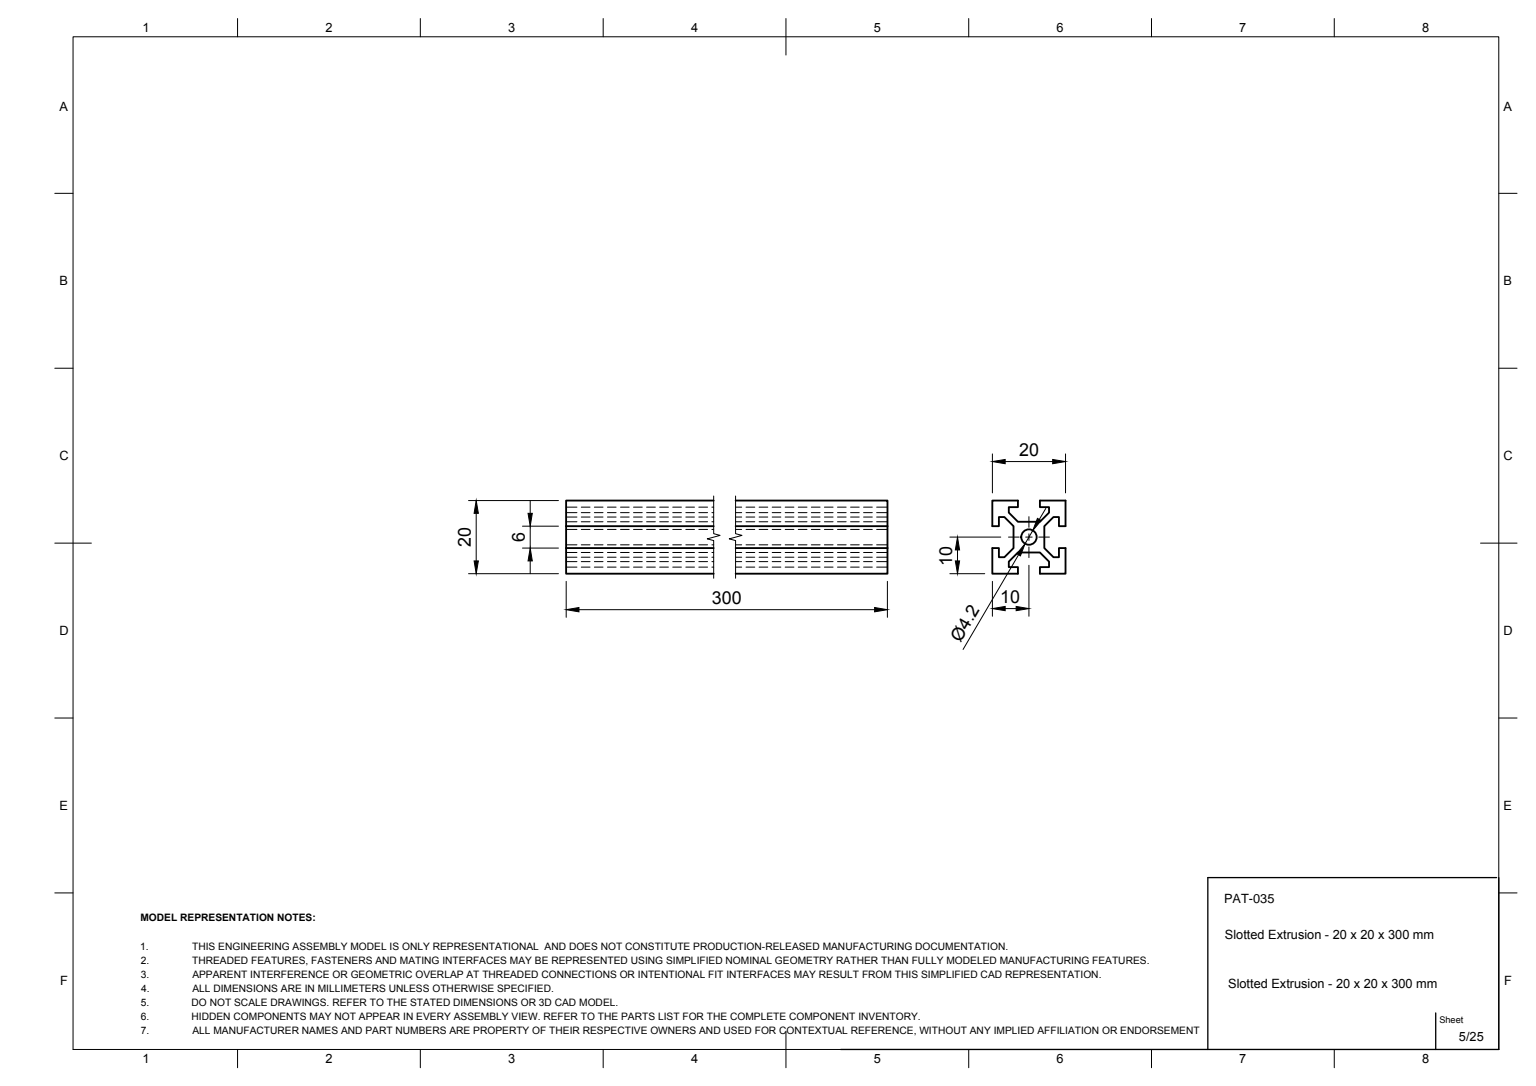
ISO-10303-21;
HEADER;
/* Generated by software containing ST-Developer
 * from STEP Tools, Inc. (www.steptools.com) 
 */

FILE_DESCRIPTION(
/* description */ ('Five-roller gravity conveyor'),
/* implementation_level */ '2;1');

FILE_NAME(
/* name */ 'Slotted Extrusion - 20 x 20 x 300 mm.step',
/* time_stamp */ '2026-10-29T15:36:43-07:00',
/* author */ (''),
/* organization */ (''),
/* preprocessor_version */ 'ST-DEVELOPER v20.2',
/* originating_system */ 'Autodesk Translation Framework v15.17.0.0',
/* authorisation */ '');

FILE_SCHEMA (('AUTOMOTIVE_DESIGN { 1 0 10303 214 3 1 1 }'));
ENDSEC;

DATA;
#10=MECHANICAL_DESIGN_GEOMETRIC_PRESENTATION_REPRESENTATION('',(#312),#7806);
#276=SHAPE_REPRESENTATION_RELATIONSHIP('SRR','None',#7912,#294);
#294=ADVANCED_BREP_SHAPE_REPRESENTATION('',(#338),#7785);
#312=STYLED_ITEM('',(#8105),#338);
#338=MANIFOLD_SOLID_BREP('Body1',#4199);
#362=FACE_BOUND('',#930,.T.);
#363=FACE_BOUND('',#932,.T.);
#421=CIRCLE('',#4466,0.21);
#422=CIRCLE('',#4467,0.21);
#594=CYLINDRICAL_SURFACE('',#4465,0.21);
#652=FACE_OUTER_BOUND('',#884,.T.);
#653=FACE_OUTER_BOUND('',#885,.T.);
#654=FACE_OUTER_BOUND('',#886,.T.);
#655=FACE_OUTER_BOUND('',#887,.T.);
#656=FACE_OUTER_BOUND('',#888,.T.);
#657=FACE_OUTER_BOUND('',#889,.T.);
#658=FACE_OUTER_BOUND('',#890,.T.);
#659=FACE_OUTER_BOUND('',#891,.T.);
#660=FACE_OUTER_BOUND('',#892,.T.);
#661=FACE_OUTER_BOUND('',#893,.T.);
#662=FACE_OUTER_BOUND('',#894,.T.);
#663=FACE_OUTER_BOUND('',#895,.T.);
#664=FACE_OUTER_BOUND('',#896,.T.);
#665=FACE_OUTER_BOUND('',#897,.T.);
#666=FACE_OUTER_BOUND('',#898,.T.);
#667=FACE_OUTER_BOUND('',#899,.T.);
#668=FACE_OUTER_BOUND('',#900,.T.);
#669=FACE_OUTER_BOUND('',#901,.T.);
#670=FACE_OUTER_BOUND('',#902,.T.);
#671=FACE_OUTER_BOUND('',#903,.T.);
#672=FACE_OUTER_BOUND('',#904,.T.);
#673=FACE_OUTER_BOUND('',#905,.T.);
#674=FACE_OUTER_BOUND('',#906,.T.);
#675=FACE_OUTER_BOUND('',#907,.T.);
#676=FACE_OUTER_BOUND('',#908,.T.);
#677=FACE_OUTER_BOUND('',#909,.T.);
#678=FACE_OUTER_BOUND('',#910,.T.);
#679=FACE_OUTER_BOUND('',#911,.T.);
#680=FACE_OUTER_BOUND('',#912,.T.);
#681=FACE_OUTER_BOUND('',#913,.T.);
#682=FACE_OUTER_BOUND('',#914,.T.);
#683=FACE_OUTER_BOUND('',#915,.T.);
#684=FACE_OUTER_BOUND('',#916,.T.);
#685=FACE_OUTER_BOUND('',#917,.T.);
#686=FACE_OUTER_BOUND('',#918,.T.);
#687=FACE_OUTER_BOUND('',#919,.T.);
#688=FACE_OUTER_BOUND('',#920,.T.);
#689=FACE_OUTER_BOUND('',#921,.T.);
#690=FACE_OUTER_BOUND('',#922,.T.);
#691=FACE_OUTER_BOUND('',#923,.T.);
#692=FACE_OUTER_BOUND('',#924,.T.);
#693=FACE_OUTER_BOUND('',#925,.T.);
#694=FACE_OUTER_BOUND('',#926,.T.);
#695=FACE_OUTER_BOUND('',#927,.T.);
#696=FACE_OUTER_BOUND('',#928,.T.);
#697=FACE_OUTER_BOUND('',#929,.T.);
#698=FACE_OUTER_BOUND('',#931,.T.);
#884=EDGE_LOOP('',(#2754,#2755,#2756,#2757));
#885=EDGE_LOOP('',(#2758,#2759,#2760,#2761));
#886=EDGE_LOOP('',(#2762,#2763,#2764,#2765));
#887=EDGE_LOOP('',(#2766,#2767,#2768,#2769));
#888=EDGE_LOOP('',(#2770,#2771,#2772,#2773));
#889=EDGE_LOOP('',(#2774,#2775,#2776,#2777));
#890=EDGE_LOOP('',(#2778,#2779,#2780,#2781));
#891=EDGE_LOOP('',(#2782,#2783,#2784,#2785));
#892=EDGE_LOOP('',(#2786,#2787,#2788,#2789));
#893=EDGE_LOOP('',(#2790,#2791,#2792,#2793));
#894=EDGE_LOOP('',(#2794,#2795,#2796,#2797));
#895=EDGE_LOOP('',(#2798,#2799,#2800,#2801));
#896=EDGE_LOOP('',(#2802,#2803,#2804,#2805));
#897=EDGE_LOOP('',(#2806,#2807,#2808,#2809));
#898=EDGE_LOOP('',(#2810,#2811,#2812,#2813));
#899=EDGE_LOOP('',(#2814,#2815,#2816,#2817));
#900=EDGE_LOOP('',(#2818,#2819,#2820,#2821));
#901=EDGE_LOOP('',(#2822,#2823,#2824,#2825));
#902=EDGE_LOOP('',(#2826,#2827,#2828,#2829));
#903=EDGE_LOOP('',(#2830,#2831,#2832,#2833));
#904=EDGE_LOOP('',(#2834,#2835,#2836,#2837));
#905=EDGE_LOOP('',(#2838,#2839,#2840,#2841));
#906=EDGE_LOOP('',(#2842,#2843,#2844,#2845));
#907=EDGE_LOOP('',(#2846,#2847,#2848,#2849));
#908=EDGE_LOOP('',(#2850,#2851,#2852,#2853));
#909=EDGE_LOOP('',(#2854,#2855,#2856,#2857));
#910=EDGE_LOOP('',(#2858,#2859,#2860,#2861));
#911=EDGE_LOOP('',(#2862,#2863,#2864,#2865));
#912=EDGE_LOOP('',(#2866,#2867,#2868,#2869));
#913=EDGE_LOOP('',(#2870,#2871,#2872,#2873));
#914=EDGE_LOOP('',(#2874,#2875,#2876,#2877));
#915=EDGE_LOOP('',(#2878,#2879,#2880,#2881));
#916=EDGE_LOOP('',(#2882,#2883,#2884,#2885));
#917=EDGE_LOOP('',(#2886,#2887,#2888,#2889));
#918=EDGE_LOOP('',(#2890,#2891,#2892,#2893));
#919=EDGE_LOOP('',(#2894,#2895,#2896,#2897));
#920=EDGE_LOOP('',(#2898,#2899,#2900,#2901));
#921=EDGE_LOOP('',(#2902,#2903,#2904,#2905));
#922=EDGE_LOOP('',(#2906,#2907,#2908,#2909));
#923=EDGE_LOOP('',(#2910,#2911,#2912,#2913));
#924=EDGE_LOOP('',(#2914,#2915,#2916,#2917));
#925=EDGE_LOOP('',(#2918,#2919,#2920,#2921));
#926=EDGE_LOOP('',(#2922,#2923,#2924,#2925));
#927=EDGE_LOOP('',(#2926,#2927,#2928,#2929));
#928=EDGE_LOOP('',(#2930,#2931,#2932,#2933));
#929=EDGE_LOOP('',(#2934,#2935,#2936,#2937,#2938,#2939,#2940,#2941,#2942,
#2943,#2944,#2945,#2946,#2947,#2948,#2949,#2950,#2951,#2952,#2953,#2954,
#2955,#2956,#2957,#2958,#2959,#2960,#2961,#2962,#2963,#2964,#2965,#2966,
#2967,#2968,#2969,#2970,#2971,#2972,#2973,#2974,#2975,#2976,#2977));
#930=EDGE_LOOP('',(#2978));
#931=EDGE_LOOP('',(#2979,#2980,#2981,#2982,#2983,#2984,#2985,#2986,#2987,
#2988,#2989,#2990,#2991,#2992,#2993,#2994,#2995,#2996,#2997,#2998,#2999,
#3000,#3001,#3002,#3003,#3004,#3005,#3006,#3007,#3008,#3009,#3010,#3011,
#3012,#3013,#3014,#3015,#3016,#3017,#3018,#3019,#3020,#3021,#3022));
#932=EDGE_LOOP('',(#3023));
#1175=LINE('',#6222,#1516);
#1176=LINE('',#6224,#1517);
#1177=LINE('',#6226,#1518);
#1178=LINE('',#6227,#1519);
#1179=LINE('',#6230,#1520);
#1180=LINE('',#6232,#1521);
#1181=LINE('',#6233,#1522);
#1182=LINE('',#6236,#1523);
#1183=LINE('',#6238,#1524);
#1184=LINE('',#6239,#1525);
#1185=LINE('',#6242,#1526);
#1186=LINE('',#6244,#1527);
#1187=LINE('',#6245,#1528);
#1188=LINE('',#6248,#1529);
#1189=LINE('',#6250,#1530);
#1190=LINE('',#6251,#1531);
#1191=LINE('',#6254,#1532);
#1192=LINE('',#6256,#1533);
#1193=LINE('',#6257,#1534);
#1194=LINE('',#6260,#1535);
#1195=LINE('',#6262,#1536);
#1196=LINE('',#6263,#1537);
#1197=LINE('',#6266,#1538);
#1198=LINE('',#6268,#1539);
#1199=LINE('',#6269,#1540);
#1200=LINE('',#6272,#1541);
#1201=LINE('',#6274,#1542);
#1202=LINE('',#6275,#1543);
#1203=LINE('',#6279,#1544);
#1204=LINE('',#6281,#1545);
#1205=LINE('',#6283,#1546);
#1206=LINE('',#6284,#1547);
#1207=LINE('',#6287,#1548);
#1208=LINE('',#6289,#1549);
#1209=LINE('',#6290,#1550);
#1210=LINE('',#6293,#1551);
#1211=LINE('',#6295,#1552);
#1212=LINE('',#6296,#1553);
#1213=LINE('',#6299,#1554);
#1214=LINE('',#6301,#1555);
#1215=LINE('',#6302,#1556);
#1216=LINE('',#6305,#1557);
#1217=LINE('',#6307,#1558);
#1218=LINE('',#6308,#1559);
#1219=LINE('',#6311,#1560);
#1220=LINE('',#6313,#1561);
#1221=LINE('',#6314,#1562);
#1222=LINE('',#6317,#1563);
#1223=LINE('',#6319,#1564);
#1224=LINE('',#6320,#1565);
#1225=LINE('',#6323,#1566);
#1226=LINE('',#6325,#1567);
#1227=LINE('',#6326,#1568);
#1228=LINE('',#6329,#1569);
#1229=LINE('',#6331,#1570);
#1230=LINE('',#6332,#1571);
#1231=LINE('',#6336,#1572);
#1232=LINE('',#6338,#1573);
#1233=LINE('',#6340,#1574);
#1234=LINE('',#6341,#1575);
#1235=LINE('',#6344,#1576);
#1236=LINE('',#6346,#1577);
#1237=LINE('',#6347,#1578);
#1238=LINE('',#6350,#1579);
#1239=LINE('',#6352,#1580);
#1240=LINE('',#6353,#1581);
#1241=LINE('',#6356,#1582);
#1242=LINE('',#6358,#1583);
#1243=LINE('',#6359,#1584);
#1244=LINE('',#6362,#1585);
#1245=LINE('',#6364,#1586);
#1246=LINE('',#6365,#1587);
#1247=LINE('',#6368,#1588);
#1248=LINE('',#6370,#1589);
#1249=LINE('',#6371,#1590);
#1250=LINE('',#6374,#1591);
#1251=LINE('',#6376,#1592);
#1252=LINE('',#6377,#1593);
#1253=LINE('',#6380,#1594);
#1254=LINE('',#6382,#1595);
#1255=LINE('',#6383,#1596);
#1256=LINE('',#6386,#1597);
#1257=LINE('',#6388,#1598);
#1258=LINE('',#6389,#1599);
#1259=LINE('',#6393,#1600);
#1260=LINE('',#6395,#1601);
#1261=LINE('',#6397,#1602);
#1262=LINE('',#6398,#1603);
#1263=LINE('',#6401,#1604);
#1264=LINE('',#6403,#1605);
#1265=LINE('',#6404,#1606);
#1266=LINE('',#6407,#1607);
#1267=LINE('',#6409,#1608);
#1268=LINE('',#6410,#1609);
#1269=LINE('',#6413,#1610);
#1270=LINE('',#6415,#1611);
#1271=LINE('',#6416,#1612);
#1272=LINE('',#6419,#1613);
#1273=LINE('',#6421,#1614);
#1274=LINE('',#6422,#1615);
#1275=LINE('',#6425,#1616);
#1276=LINE('',#6427,#1617);
#1277=LINE('',#6428,#1618);
#1278=LINE('',#6431,#1619);
#1279=LINE('',#6433,#1620);
#1280=LINE('',#6434,#1621);
#1281=LINE('',#6437,#1622);
#1282=LINE('',#6439,#1623);
#1283=LINE('',#6440,#1624);
#1284=LINE('',#6443,#1625);
#1285=LINE('',#6445,#1626);
#1286=LINE('',#6446,#1627);
#1287=LINE('',#6451,#1628);
#1288=LINE('',#6455,#1629);
#1289=LINE('',#6457,#1630);
#1290=LINE('',#6458,#1631);
#1291=LINE('',#6461,#1632);
#1292=LINE('',#6463,#1633);
#1293=LINE('',#6464,#1634);
#1294=LINE('',#6466,#1635);
#1295=LINE('',#6467,#1636);
#1296=LINE('',#6470,#1637);
#1297=LINE('',#6472,#1638);
#1298=LINE('',#6473,#1639);
#1299=LINE('',#6475,#1640);
#1300=LINE('',#6476,#1641);
#1301=LINE('',#6479,#1642);
#1302=LINE('',#6481,#1643);
#1303=LINE('',#6482,#1644);
#1304=LINE('',#6484,#1645);
#1305=LINE('',#6485,#1646);
#1306=LINE('',#6487,#1647);
#1307=LINE('',#6488,#1648);
#1516=VECTOR('',#4917,1.);
#1517=VECTOR('',#4918,1.);
#1518=VECTOR('',#4919,1.);
#1519=VECTOR('',#4920,1.);
#1520=VECTOR('',#4923,1.);
#1521=VECTOR('',#4924,1.);
#1522=VECTOR('',#4925,1.);
#1523=VECTOR('',#4928,1.);
#1524=VECTOR('',#4929,1.);
#1525=VECTOR('',#4930,1.);
#1526=VECTOR('',#4933,1.);
#1527=VECTOR('',#4934,1.);
#1528=VECTOR('',#4935,1.);
#1529=VECTOR('',#4938,1.);
#1530=VECTOR('',#4939,1.);
#1531=VECTOR('',#4940,1.);
#1532=VECTOR('',#4943,1.);
#1533=VECTOR('',#4944,1.);
#1534=VECTOR('',#4945,1.);
#1535=VECTOR('',#4948,1.);
#1536=VECTOR('',#4949,1.);
#1537=VECTOR('',#4950,1.);
#1538=VECTOR('',#4953,1.);
#1539=VECTOR('',#4954,1.);
#1540=VECTOR('',#4955,1.);
#1541=VECTOR('',#4958,1.);
#1542=VECTOR('',#4959,1.);
#1543=VECTOR('',#4960,1.);
#1544=VECTOR('',#4963,1.);
#1545=VECTOR('',#4964,1.);
#1546=VECTOR('',#4965,1.);
#1547=VECTOR('',#4966,1.);
#1548=VECTOR('',#4969,1.);
#1549=VECTOR('',#4970,1.);
#1550=VECTOR('',#4971,1.);
#1551=VECTOR('',#4974,1.);
#1552=VECTOR('',#4975,1.);
#1553=VECTOR('',#4976,1.);
#1554=VECTOR('',#4979,1.);
#1555=VECTOR('',#4980,1.);
#1556=VECTOR('',#4981,1.);
#1557=VECTOR('',#4984,1.);
#1558=VECTOR('',#4985,1.);
#1559=VECTOR('',#4986,1.);
#1560=VECTOR('',#4989,1.);
#1561=VECTOR('',#4990,1.);
#1562=VECTOR('',#4991,1.);
#1563=VECTOR('',#4994,1.);
#1564=VECTOR('',#4995,1.);
#1565=VECTOR('',#4996,1.);
#1566=VECTOR('',#4999,1.);
#1567=VECTOR('',#5000,1.);
#1568=VECTOR('',#5001,1.);
#1569=VECTOR('',#5004,1.);
#1570=VECTOR('',#5005,1.);
#1571=VECTOR('',#5006,1.);
#1572=VECTOR('',#5009,1.);
#1573=VECTOR('',#5010,1.);
#1574=VECTOR('',#5011,1.);
#1575=VECTOR('',#5012,1.);
#1576=VECTOR('',#5015,1.);
#1577=VECTOR('',#5016,1.);
#1578=VECTOR('',#5017,1.);
#1579=VECTOR('',#5020,1.);
#1580=VECTOR('',#5021,1.);
#1581=VECTOR('',#5022,1.);
#1582=VECTOR('',#5025,1.);
#1583=VECTOR('',#5026,1.);
#1584=VECTOR('',#5027,1.);
#1585=VECTOR('',#5030,1.);
#1586=VECTOR('',#5031,1.);
#1587=VECTOR('',#5032,1.);
#1588=VECTOR('',#5035,1.);
#1589=VECTOR('',#5036,1.);
#1590=VECTOR('',#5037,1.);
#1591=VECTOR('',#5040,1.);
#1592=VECTOR('',#5041,1.);
#1593=VECTOR('',#5042,1.);
#1594=VECTOR('',#5045,1.);
#1595=VECTOR('',#5046,1.);
#1596=VECTOR('',#5047,1.);
#1597=VECTOR('',#5050,1.);
#1598=VECTOR('',#5051,1.);
#1599=VECTOR('',#5052,1.);
#1600=VECTOR('',#5055,1.);
#1601=VECTOR('',#5056,1.);
#1602=VECTOR('',#5057,1.);
#1603=VECTOR('',#5058,1.);
#1604=VECTOR('',#5061,1.);
#1605=VECTOR('',#5062,1.);
#1606=VECTOR('',#5063,1.);
#1607=VECTOR('',#5066,1.);
#1608=VECTOR('',#5067,1.);
#1609=VECTOR('',#5068,1.);
#1610=VECTOR('',#5071,1.);
#1611=VECTOR('',#5072,1.);
#1612=VECTOR('',#5073,1.);
#1613=VECTOR('',#5076,1.);
#1614=VECTOR('',#5077,1.);
#1615=VECTOR('',#5078,1.);
#1616=VECTOR('',#5081,1.);
#1617=VECTOR('',#5082,1.);
#1618=VECTOR('',#5083,1.);
#1619=VECTOR('',#5086,1.);
#1620=VECTOR('',#5087,1.);
#1621=VECTOR('',#5088,1.);
#1622=VECTOR('',#5091,1.);
#1623=VECTOR('',#5092,1.);
#1624=VECTOR('',#5093,1.);
#1625=VECTOR('',#5096,1.);
#1626=VECTOR('',#5097,1.);
#1627=VECTOR('',#5098,1.);
#1628=VECTOR('',#5103,0.21);
#1629=VECTOR('',#5108,1.);
#1630=VECTOR('',#5109,1.);
#1631=VECTOR('',#5110,1.);
#1632=VECTOR('',#5113,1.);
#1633=VECTOR('',#5114,1.);
#1634=VECTOR('',#5115,1.);
#1635=VECTOR('',#5118,1.);
#1636=VECTOR('',#5119,1.);
#1637=VECTOR('',#5122,1.);
#1638=VECTOR('',#5123,1.);
#1639=VECTOR('',#5124,1.);
#1640=VECTOR('',#5127,1.);
#1641=VECTOR('',#5128,1.);
#1642=VECTOR('',#5131,1.);
#1643=VECTOR('',#5132,1.);
#1644=VECTOR('',#5133,1.);
#1645=VECTOR('',#5136,1.);
#1646=VECTOR('',#5137,1.);
#1647=VECTOR('',#5140,1.);
#1648=VECTOR('',#5141,1.);
#1857=VERTEX_POINT('',#6220);
#1858=VERTEX_POINT('',#6221);
#1859=VERTEX_POINT('',#6223);
#1860=VERTEX_POINT('',#6225);
#1861=VERTEX_POINT('',#6229);
#1862=VERTEX_POINT('',#6231);
#1863=VERTEX_POINT('',#6235);
#1864=VERTEX_POINT('',#6237);
#1865=VERTEX_POINT('',#6241);
#1866=VERTEX_POINT('',#6243);
#1867=VERTEX_POINT('',#6247);
#1868=VERTEX_POINT('',#6249);
#1869=VERTEX_POINT('',#6253);
#1870=VERTEX_POINT('',#6255);
#1871=VERTEX_POINT('',#6259);
#1872=VERTEX_POINT('',#6261);
#1873=VERTEX_POINT('',#6265);
#1874=VERTEX_POINT('',#6267);
#1875=VERTEX_POINT('',#6271);
#1876=VERTEX_POINT('',#6273);
#1877=VERTEX_POINT('',#6277);
#1878=VERTEX_POINT('',#6278);
#1879=VERTEX_POINT('',#6280);
#1880=VERTEX_POINT('',#6282);
#1881=VERTEX_POINT('',#6286);
#1882=VERTEX_POINT('',#6288);
#1883=VERTEX_POINT('',#6292);
#1884=VERTEX_POINT('',#6294);
#1885=VERTEX_POINT('',#6298);
#1886=VERTEX_POINT('',#6300);
#1887=VERTEX_POINT('',#6304);
#1888=VERTEX_POINT('',#6306);
#1889=VERTEX_POINT('',#6310);
#1890=VERTEX_POINT('',#6312);
#1891=VERTEX_POINT('',#6316);
#1892=VERTEX_POINT('',#6318);
#1893=VERTEX_POINT('',#6322);
#1894=VERTEX_POINT('',#6324);
#1895=VERTEX_POINT('',#6328);
#1896=VERTEX_POINT('',#6330);
#1897=VERTEX_POINT('',#6334);
#1898=VERTEX_POINT('',#6335);
#1899=VERTEX_POINT('',#6337);
#1900=VERTEX_POINT('',#6339);
#1901=VERTEX_POINT('',#6343);
#1902=VERTEX_POINT('',#6345);
#1903=VERTEX_POINT('',#6349);
#1904=VERTEX_POINT('',#6351);
#1905=VERTEX_POINT('',#6355);
#1906=VERTEX_POINT('',#6357);
#1907=VERTEX_POINT('',#6361);
#1908=VERTEX_POINT('',#6363);
#1909=VERTEX_POINT('',#6367);
#1910=VERTEX_POINT('',#6369);
#1911=VERTEX_POINT('',#6373);
#1912=VERTEX_POINT('',#6375);
#1913=VERTEX_POINT('',#6379);
#1914=VERTEX_POINT('',#6381);
#1915=VERTEX_POINT('',#6385);
#1916=VERTEX_POINT('',#6387);
#1917=VERTEX_POINT('',#6391);
#1918=VERTEX_POINT('',#6392);
#1919=VERTEX_POINT('',#6394);
#1920=VERTEX_POINT('',#6396);
#1921=VERTEX_POINT('',#6400);
#1922=VERTEX_POINT('',#6402);
#1923=VERTEX_POINT('',#6406);
#1924=VERTEX_POINT('',#6408);
#1925=VERTEX_POINT('',#6412);
#1926=VERTEX_POINT('',#6414);
#1927=VERTEX_POINT('',#6418);
#1928=VERTEX_POINT('',#6420);
#1929=VERTEX_POINT('',#6424);
#1930=VERTEX_POINT('',#6426);
#1931=VERTEX_POINT('',#6430);
#1932=VERTEX_POINT('',#6432);
#1933=VERTEX_POINT('',#6436);
#1934=VERTEX_POINT('',#6438);
#1935=VERTEX_POINT('',#6442);
#1936=VERTEX_POINT('',#6444);
#1937=VERTEX_POINT('',#6448);
#1938=VERTEX_POINT('',#6450);
#1939=VERTEX_POINT('',#6454);
#1940=VERTEX_POINT('',#6456);
#1941=VERTEX_POINT('',#6460);
#1942=VERTEX_POINT('',#6462);
#1943=VERTEX_POINT('',#6469);
#1944=VERTEX_POINT('',#6471);
#1945=VERTEX_POINT('',#6478);
#1946=VERTEX_POINT('',#6480);
#2220=EDGE_CURVE('',#1857,#1858,#1175,.T.);
#2221=EDGE_CURVE('',#1857,#1859,#1176,.T.);
#2222=EDGE_CURVE('',#1860,#1859,#1177,.T.);
#2223=EDGE_CURVE('',#1858,#1860,#1178,.T.);
#2224=EDGE_CURVE('',#1861,#1857,#1179,.T.);
#2225=EDGE_CURVE('',#1861,#1862,#1180,.T.);
#2226=EDGE_CURVE('',#1859,#1862,#1181,.T.);
#2227=EDGE_CURVE('',#1863,#1861,#1182,.T.);
#2228=EDGE_CURVE('',#1863,#1864,#1183,.T.);
#2229=EDGE_CURVE('',#1862,#1864,#1184,.T.);
#2230=EDGE_CURVE('',#1865,#1863,#1185,.T.);
#2231=EDGE_CURVE('',#1865,#1866,#1186,.T.);
#2232=EDGE_CURVE('',#1864,#1866,#1187,.T.);
#2233=EDGE_CURVE('',#1867,#1865,#1188,.T.);
#2234=EDGE_CURVE('',#1867,#1868,#1189,.T.);
#2235=EDGE_CURVE('',#1866,#1868,#1190,.T.);
#2236=EDGE_CURVE('',#1869,#1867,#1191,.T.);
#2237=EDGE_CURVE('',#1869,#1870,#1192,.T.);
#2238=EDGE_CURVE('',#1868,#1870,#1193,.T.);
#2239=EDGE_CURVE('',#1871,#1869,#1194,.T.);
#2240=EDGE_CURVE('',#1871,#1872,#1195,.T.);
#2241=EDGE_CURVE('',#1870,#1872,#1196,.T.);
#2242=EDGE_CURVE('',#1873,#1871,#1197,.T.);
#2243=EDGE_CURVE('',#1873,#1874,#1198,.T.);
#2244=EDGE_CURVE('',#1872,#1874,#1199,.T.);
#2245=EDGE_CURVE('',#1875,#1873,#1200,.T.);
#2246=EDGE_CURVE('',#1876,#1875,#1201,.T.);
#2247=EDGE_CURVE('',#1874,#1876,#1202,.T.);
#2248=EDGE_CURVE('',#1877,#1878,#1203,.T.);
#2249=EDGE_CURVE('',#1877,#1879,#1204,.T.);
#2250=EDGE_CURVE('',#1880,#1879,#1205,.T.);
#2251=EDGE_CURVE('',#1878,#1880,#1206,.T.);
#2252=EDGE_CURVE('',#1881,#1877,#1207,.T.);
#2253=EDGE_CURVE('',#1881,#1882,#1208,.T.);
#2254=EDGE_CURVE('',#1879,#1882,#1209,.T.);
#2255=EDGE_CURVE('',#1883,#1881,#1210,.T.);
#2256=EDGE_CURVE('',#1883,#1884,#1211,.T.);
#2257=EDGE_CURVE('',#1882,#1884,#1212,.T.);
#2258=EDGE_CURVE('',#1885,#1883,#1213,.T.);
#2259=EDGE_CURVE('',#1885,#1886,#1214,.T.);
#2260=EDGE_CURVE('',#1884,#1886,#1215,.T.);
#2261=EDGE_CURVE('',#1887,#1885,#1216,.T.);
#2262=EDGE_CURVE('',#1887,#1888,#1217,.T.);
#2263=EDGE_CURVE('',#1886,#1888,#1218,.T.);
#2264=EDGE_CURVE('',#1889,#1887,#1219,.T.);
#2265=EDGE_CURVE('',#1889,#1890,#1220,.T.);
#2266=EDGE_CURVE('',#1888,#1890,#1221,.T.);
#2267=EDGE_CURVE('',#1891,#1889,#1222,.T.);
#2268=EDGE_CURVE('',#1891,#1892,#1223,.T.);
#2269=EDGE_CURVE('',#1890,#1892,#1224,.T.);
#2270=EDGE_CURVE('',#1893,#1891,#1225,.T.);
#2271=EDGE_CURVE('',#1893,#1894,#1226,.T.);
#2272=EDGE_CURVE('',#1892,#1894,#1227,.T.);
#2273=EDGE_CURVE('',#1895,#1893,#1228,.T.);
#2274=EDGE_CURVE('',#1896,#1895,#1229,.T.);
#2275=EDGE_CURVE('',#1894,#1896,#1230,.T.);
#2276=EDGE_CURVE('',#1897,#1898,#1231,.T.);
#2277=EDGE_CURVE('',#1897,#1899,#1232,.T.);
#2278=EDGE_CURVE('',#1900,#1899,#1233,.T.);
#2279=EDGE_CURVE('',#1898,#1900,#1234,.T.);
#2280=EDGE_CURVE('',#1901,#1897,#1235,.T.);
#2281=EDGE_CURVE('',#1901,#1902,#1236,.T.);
#2282=EDGE_CURVE('',#1899,#1902,#1237,.T.);
#2283=EDGE_CURVE('',#1903,#1901,#1238,.T.);
#2284=EDGE_CURVE('',#1903,#1904,#1239,.T.);
#2285=EDGE_CURVE('',#1902,#1904,#1240,.T.);
#2286=EDGE_CURVE('',#1905,#1903,#1241,.T.);
#2287=EDGE_CURVE('',#1905,#1906,#1242,.T.);
#2288=EDGE_CURVE('',#1904,#1906,#1243,.T.);
#2289=EDGE_CURVE('',#1907,#1905,#1244,.T.);
#2290=EDGE_CURVE('',#1907,#1908,#1245,.T.);
#2291=EDGE_CURVE('',#1906,#1908,#1246,.T.);
#2292=EDGE_CURVE('',#1909,#1907,#1247,.T.);
#2293=EDGE_CURVE('',#1909,#1910,#1248,.T.);
#2294=EDGE_CURVE('',#1908,#1910,#1249,.T.);
#2295=EDGE_CURVE('',#1911,#1909,#1250,.T.);
#2296=EDGE_CURVE('',#1911,#1912,#1251,.T.);
#2297=EDGE_CURVE('',#1910,#1912,#1252,.T.);
#2298=EDGE_CURVE('',#1913,#1911,#1253,.T.);
#2299=EDGE_CURVE('',#1913,#1914,#1254,.T.);
#2300=EDGE_CURVE('',#1912,#1914,#1255,.T.);
#2301=EDGE_CURVE('',#1915,#1913,#1256,.T.);
#2302=EDGE_CURVE('',#1916,#1915,#1257,.T.);
#2303=EDGE_CURVE('',#1914,#1916,#1258,.T.);
#2304=EDGE_CURVE('',#1917,#1918,#1259,.T.);
#2305=EDGE_CURVE('',#1917,#1919,#1260,.T.);
#2306=EDGE_CURVE('',#1920,#1919,#1261,.T.);
#2307=EDGE_CURVE('',#1918,#1920,#1262,.T.);
#2308=EDGE_CURVE('',#1921,#1917,#1263,.T.);
#2309=EDGE_CURVE('',#1921,#1922,#1264,.T.);
#2310=EDGE_CURVE('',#1919,#1922,#1265,.T.);
#2311=EDGE_CURVE('',#1923,#1921,#1266,.T.);
#2312=EDGE_CURVE('',#1923,#1924,#1267,.T.);
#2313=EDGE_CURVE('',#1922,#1924,#1268,.T.);
#2314=EDGE_CURVE('',#1925,#1923,#1269,.T.);
#2315=EDGE_CURVE('',#1925,#1926,#1270,.T.);
#2316=EDGE_CURVE('',#1924,#1926,#1271,.T.);
#2317=EDGE_CURVE('',#1927,#1925,#1272,.T.);
#2318=EDGE_CURVE('',#1927,#1928,#1273,.T.);
#2319=EDGE_CURVE('',#1926,#1928,#1274,.T.);
#2320=EDGE_CURVE('',#1929,#1927,#1275,.T.);
#2321=EDGE_CURVE('',#1929,#1930,#1276,.T.);
#2322=EDGE_CURVE('',#1928,#1930,#1277,.T.);
#2323=EDGE_CURVE('',#1931,#1929,#1278,.T.);
#2324=EDGE_CURVE('',#1931,#1932,#1279,.T.);
#2325=EDGE_CURVE('',#1930,#1932,#1280,.T.);
#2326=EDGE_CURVE('',#1933,#1931,#1281,.T.);
#2327=EDGE_CURVE('',#1933,#1934,#1282,.T.);
#2328=EDGE_CURVE('',#1932,#1934,#1283,.T.);
#2329=EDGE_CURVE('',#1935,#1933,#1284,.T.);
#2330=EDGE_CURVE('',#1936,#1935,#1285,.T.);
#2331=EDGE_CURVE('',#1934,#1936,#1286,.T.);
#2332=EDGE_CURVE('',#1937,#1937,#421,.T.);
#2333=EDGE_CURVE('',#1937,#1938,#1287,.T.);
#2334=EDGE_CURVE('',#1938,#1938,#422,.T.);
#2335=EDGE_CURVE('',#1875,#1939,#1288,.T.);
#2336=EDGE_CURVE('',#1939,#1940,#1289,.T.);
#2337=EDGE_CURVE('',#1876,#1940,#1290,.T.);
#2338=EDGE_CURVE('',#1941,#1860,#1291,.T.);
#2339=EDGE_CURVE('',#1942,#1941,#1292,.T.);
#2340=EDGE_CURVE('',#1942,#1858,#1293,.T.);
#2341=EDGE_CURVE('',#1895,#1942,#1294,.T.);
#2342=EDGE_CURVE('',#1896,#1941,#1295,.T.);
#2343=EDGE_CURVE('',#1943,#1880,#1296,.T.);
#2344=EDGE_CURVE('',#1944,#1943,#1297,.T.);
#2345=EDGE_CURVE('',#1944,#1878,#1298,.T.);
#2346=EDGE_CURVE('',#1915,#1944,#1299,.T.);
#2347=EDGE_CURVE('',#1916,#1943,#1300,.T.);
#2348=EDGE_CURVE('',#1945,#1900,#1301,.T.);
#2349=EDGE_CURVE('',#1946,#1945,#1302,.T.);
#2350=EDGE_CURVE('',#1946,#1898,#1303,.T.);
#2351=EDGE_CURVE('',#1935,#1946,#1304,.T.);
#2352=EDGE_CURVE('',#1936,#1945,#1305,.T.);
#2353=EDGE_CURVE('',#1940,#1920,#1306,.T.);
#2354=EDGE_CURVE('',#1939,#1918,#1307,.T.);
#2754=ORIENTED_EDGE('',*,*,#2220,.F.);
#2755=ORIENTED_EDGE('',*,*,#2221,.T.);
#2756=ORIENTED_EDGE('',*,*,#2222,.F.);
#2757=ORIENTED_EDGE('',*,*,#2223,.F.);
#2758=ORIENTED_EDGE('',*,*,#2224,.F.);
#2759=ORIENTED_EDGE('',*,*,#2225,.T.);
#2760=ORIENTED_EDGE('',*,*,#2226,.F.);
#2761=ORIENTED_EDGE('',*,*,#2221,.F.);
#2762=ORIENTED_EDGE('',*,*,#2227,.F.);
#2763=ORIENTED_EDGE('',*,*,#2228,.T.);
#2764=ORIENTED_EDGE('',*,*,#2229,.F.);
#2765=ORIENTED_EDGE('',*,*,#2225,.F.);
#2766=ORIENTED_EDGE('',*,*,#2230,.F.);
#2767=ORIENTED_EDGE('',*,*,#2231,.T.);
#2768=ORIENTED_EDGE('',*,*,#2232,.F.);
#2769=ORIENTED_EDGE('',*,*,#2228,.F.);
#2770=ORIENTED_EDGE('',*,*,#2233,.F.);
#2771=ORIENTED_EDGE('',*,*,#2234,.T.);
#2772=ORIENTED_EDGE('',*,*,#2235,.F.);
#2773=ORIENTED_EDGE('',*,*,#2231,.F.);
#2774=ORIENTED_EDGE('',*,*,#2236,.F.);
#2775=ORIENTED_EDGE('',*,*,#2237,.T.);
#2776=ORIENTED_EDGE('',*,*,#2238,.F.);
#2777=ORIENTED_EDGE('',*,*,#2234,.F.);
#2778=ORIENTED_EDGE('',*,*,#2239,.F.);
#2779=ORIENTED_EDGE('',*,*,#2240,.T.);
#2780=ORIENTED_EDGE('',*,*,#2241,.F.);
#2781=ORIENTED_EDGE('',*,*,#2237,.F.);
#2782=ORIENTED_EDGE('',*,*,#2242,.F.);
#2783=ORIENTED_EDGE('',*,*,#2243,.T.);
#2784=ORIENTED_EDGE('',*,*,#2244,.F.);
#2785=ORIENTED_EDGE('',*,*,#2240,.F.);
#2786=ORIENTED_EDGE('',*,*,#2245,.F.);
#2787=ORIENTED_EDGE('',*,*,#2246,.F.);
#2788=ORIENTED_EDGE('',*,*,#2247,.F.);
#2789=ORIENTED_EDGE('',*,*,#2243,.F.);
#2790=ORIENTED_EDGE('',*,*,#2248,.F.);
#2791=ORIENTED_EDGE('',*,*,#2249,.T.);
#2792=ORIENTED_EDGE('',*,*,#2250,.F.);
#2793=ORIENTED_EDGE('',*,*,#2251,.F.);
#2794=ORIENTED_EDGE('',*,*,#2252,.F.);
#2795=ORIENTED_EDGE('',*,*,#2253,.T.);
#2796=ORIENTED_EDGE('',*,*,#2254,.F.);
#2797=ORIENTED_EDGE('',*,*,#2249,.F.);
#2798=ORIENTED_EDGE('',*,*,#2255,.F.);
#2799=ORIENTED_EDGE('',*,*,#2256,.T.);
#2800=ORIENTED_EDGE('',*,*,#2257,.F.);
#2801=ORIENTED_EDGE('',*,*,#2253,.F.);
#2802=ORIENTED_EDGE('',*,*,#2258,.F.);
#2803=ORIENTED_EDGE('',*,*,#2259,.T.);
#2804=ORIENTED_EDGE('',*,*,#2260,.F.);
#2805=ORIENTED_EDGE('',*,*,#2256,.F.);
#2806=ORIENTED_EDGE('',*,*,#2261,.F.);
#2807=ORIENTED_EDGE('',*,*,#2262,.T.);
#2808=ORIENTED_EDGE('',*,*,#2263,.F.);
#2809=ORIENTED_EDGE('',*,*,#2259,.F.);
#2810=ORIENTED_EDGE('',*,*,#2264,.F.);
#2811=ORIENTED_EDGE('',*,*,#2265,.T.);
#2812=ORIENTED_EDGE('',*,*,#2266,.F.);
#2813=ORIENTED_EDGE('',*,*,#2262,.F.);
#2814=ORIENTED_EDGE('',*,*,#2267,.F.);
#2815=ORIENTED_EDGE('',*,*,#2268,.T.);
#2816=ORIENTED_EDGE('',*,*,#2269,.F.);
#2817=ORIENTED_EDGE('',*,*,#2265,.F.);
#2818=ORIENTED_EDGE('',*,*,#2270,.F.);
#2819=ORIENTED_EDGE('',*,*,#2271,.T.);
#2820=ORIENTED_EDGE('',*,*,#2272,.F.);
#2821=ORIENTED_EDGE('',*,*,#2268,.F.);
#2822=ORIENTED_EDGE('',*,*,#2273,.F.);
#2823=ORIENTED_EDGE('',*,*,#2274,.F.);
#2824=ORIENTED_EDGE('',*,*,#2275,.F.);
#2825=ORIENTED_EDGE('',*,*,#2271,.F.);
#2826=ORIENTED_EDGE('',*,*,#2276,.F.);
#2827=ORIENTED_EDGE('',*,*,#2277,.T.);
#2828=ORIENTED_EDGE('',*,*,#2278,.F.);
#2829=ORIENTED_EDGE('',*,*,#2279,.F.);
#2830=ORIENTED_EDGE('',*,*,#2280,.F.);
#2831=ORIENTED_EDGE('',*,*,#2281,.T.);
#2832=ORIENTED_EDGE('',*,*,#2282,.F.);
#2833=ORIENTED_EDGE('',*,*,#2277,.F.);
#2834=ORIENTED_EDGE('',*,*,#2283,.F.);
#2835=ORIENTED_EDGE('',*,*,#2284,.T.);
#2836=ORIENTED_EDGE('',*,*,#2285,.F.);
#2837=ORIENTED_EDGE('',*,*,#2281,.F.);
#2838=ORIENTED_EDGE('',*,*,#2286,.F.);
#2839=ORIENTED_EDGE('',*,*,#2287,.T.);
#2840=ORIENTED_EDGE('',*,*,#2288,.F.);
#2841=ORIENTED_EDGE('',*,*,#2284,.F.);
#2842=ORIENTED_EDGE('',*,*,#2289,.F.);
#2843=ORIENTED_EDGE('',*,*,#2290,.T.);
#2844=ORIENTED_EDGE('',*,*,#2291,.F.);
#2845=ORIENTED_EDGE('',*,*,#2287,.F.);
#2846=ORIENTED_EDGE('',*,*,#2292,.F.);
#2847=ORIENTED_EDGE('',*,*,#2293,.T.);
#2848=ORIENTED_EDGE('',*,*,#2294,.F.);
#2849=ORIENTED_EDGE('',*,*,#2290,.F.);
#2850=ORIENTED_EDGE('',*,*,#2295,.F.);
#2851=ORIENTED_EDGE('',*,*,#2296,.T.);
#2852=ORIENTED_EDGE('',*,*,#2297,.F.);
#2853=ORIENTED_EDGE('',*,*,#2293,.F.);
#2854=ORIENTED_EDGE('',*,*,#2298,.F.);
#2855=ORIENTED_EDGE('',*,*,#2299,.T.);
#2856=ORIENTED_EDGE('',*,*,#2300,.F.);
#2857=ORIENTED_EDGE('',*,*,#2296,.F.);
#2858=ORIENTED_EDGE('',*,*,#2301,.F.);
#2859=ORIENTED_EDGE('',*,*,#2302,.F.);
#2860=ORIENTED_EDGE('',*,*,#2303,.F.);
#2861=ORIENTED_EDGE('',*,*,#2299,.F.);
#2862=ORIENTED_EDGE('',*,*,#2304,.F.);
#2863=ORIENTED_EDGE('',*,*,#2305,.T.);
#2864=ORIENTED_EDGE('',*,*,#2306,.F.);
#2865=ORIENTED_EDGE('',*,*,#2307,.F.);
#2866=ORIENTED_EDGE('',*,*,#2308,.F.);
#2867=ORIENTED_EDGE('',*,*,#2309,.T.);
#2868=ORIENTED_EDGE('',*,*,#2310,.F.);
#2869=ORIENTED_EDGE('',*,*,#2305,.F.);
#2870=ORIENTED_EDGE('',*,*,#2311,.F.);
#2871=ORIENTED_EDGE('',*,*,#2312,.T.);
#2872=ORIENTED_EDGE('',*,*,#2313,.F.);
#2873=ORIENTED_EDGE('',*,*,#2309,.F.);
#2874=ORIENTED_EDGE('',*,*,#2314,.F.);
#2875=ORIENTED_EDGE('',*,*,#2315,.T.);
#2876=ORIENTED_EDGE('',*,*,#2316,.F.);
#2877=ORIENTED_EDGE('',*,*,#2312,.F.);
#2878=ORIENTED_EDGE('',*,*,#2317,.F.);
#2879=ORIENTED_EDGE('',*,*,#2318,.T.);
#2880=ORIENTED_EDGE('',*,*,#2319,.F.);
#2881=ORIENTED_EDGE('',*,*,#2315,.F.);
#2882=ORIENTED_EDGE('',*,*,#2320,.F.);
#2883=ORIENTED_EDGE('',*,*,#2321,.T.);
#2884=ORIENTED_EDGE('',*,*,#2322,.F.);
#2885=ORIENTED_EDGE('',*,*,#2318,.F.);
#2886=ORIENTED_EDGE('',*,*,#2323,.F.);
#2887=ORIENTED_EDGE('',*,*,#2324,.T.);
#2888=ORIENTED_EDGE('',*,*,#2325,.F.);
#2889=ORIENTED_EDGE('',*,*,#2321,.F.);
#2890=ORIENTED_EDGE('',*,*,#2326,.F.);
#2891=ORIENTED_EDGE('',*,*,#2327,.T.);
#2892=ORIENTED_EDGE('',*,*,#2328,.F.);
#2893=ORIENTED_EDGE('',*,*,#2324,.F.);
#2894=ORIENTED_EDGE('',*,*,#2329,.F.);
#2895=ORIENTED_EDGE('',*,*,#2330,.F.);
#2896=ORIENTED_EDGE('',*,*,#2331,.F.);
#2897=ORIENTED_EDGE('',*,*,#2327,.F.);
#2898=ORIENTED_EDGE('',*,*,#2332,.F.);
#2899=ORIENTED_EDGE('',*,*,#2333,.T.);
#2900=ORIENTED_EDGE('',*,*,#2334,.F.);
#2901=ORIENTED_EDGE('',*,*,#2333,.F.);
#2902=ORIENTED_EDGE('',*,*,#2246,.T.);
#2903=ORIENTED_EDGE('',*,*,#2335,.T.);
#2904=ORIENTED_EDGE('',*,*,#2336,.T.);
#2905=ORIENTED_EDGE('',*,*,#2337,.F.);
#2906=ORIENTED_EDGE('',*,*,#2223,.T.);
#2907=ORIENTED_EDGE('',*,*,#2338,.F.);
#2908=ORIENTED_EDGE('',*,*,#2339,.F.);
#2909=ORIENTED_EDGE('',*,*,#2340,.T.);
#2910=ORIENTED_EDGE('',*,*,#2274,.T.);
#2911=ORIENTED_EDGE('',*,*,#2341,.T.);
#2912=ORIENTED_EDGE('',*,*,#2339,.T.);
#2913=ORIENTED_EDGE('',*,*,#2342,.F.);
#2914=ORIENTED_EDGE('',*,*,#2251,.T.);
#2915=ORIENTED_EDGE('',*,*,#2343,.F.);
#2916=ORIENTED_EDGE('',*,*,#2344,.F.);
#2917=ORIENTED_EDGE('',*,*,#2345,.T.);
#2918=ORIENTED_EDGE('',*,*,#2302,.T.);
#2919=ORIENTED_EDGE('',*,*,#2346,.T.);
#2920=ORIENTED_EDGE('',*,*,#2344,.T.);
#2921=ORIENTED_EDGE('',*,*,#2347,.F.);
#2922=ORIENTED_EDGE('',*,*,#2279,.T.);
#2923=ORIENTED_EDGE('',*,*,#2348,.F.);
#2924=ORIENTED_EDGE('',*,*,#2349,.F.);
#2925=ORIENTED_EDGE('',*,*,#2350,.T.);
#2926=ORIENTED_EDGE('',*,*,#2330,.T.);
#2927=ORIENTED_EDGE('',*,*,#2351,.T.);
#2928=ORIENTED_EDGE('',*,*,#2349,.T.);
#2929=ORIENTED_EDGE('',*,*,#2352,.F.);
#2930=ORIENTED_EDGE('',*,*,#2307,.T.);
#2931=ORIENTED_EDGE('',*,*,#2353,.F.);
#2932=ORIENTED_EDGE('',*,*,#2336,.F.);
#2933=ORIENTED_EDGE('',*,*,#2354,.T.);
#2934=ORIENTED_EDGE('',*,*,#2222,.T.);
#2935=ORIENTED_EDGE('',*,*,#2226,.T.);
#2936=ORIENTED_EDGE('',*,*,#2229,.T.);
#2937=ORIENTED_EDGE('',*,*,#2232,.T.);
#2938=ORIENTED_EDGE('',*,*,#2235,.T.);
#2939=ORIENTED_EDGE('',*,*,#2238,.T.);
#2940=ORIENTED_EDGE('',*,*,#2241,.T.);
#2941=ORIENTED_EDGE('',*,*,#2244,.T.);
#2942=ORIENTED_EDGE('',*,*,#2247,.T.);
#2943=ORIENTED_EDGE('',*,*,#2337,.T.);
#2944=ORIENTED_EDGE('',*,*,#2353,.T.);
#2945=ORIENTED_EDGE('',*,*,#2306,.T.);
#2946=ORIENTED_EDGE('',*,*,#2310,.T.);
#2947=ORIENTED_EDGE('',*,*,#2313,.T.);
#2948=ORIENTED_EDGE('',*,*,#2316,.T.);
#2949=ORIENTED_EDGE('',*,*,#2319,.T.);
#2950=ORIENTED_EDGE('',*,*,#2322,.T.);
#2951=ORIENTED_EDGE('',*,*,#2325,.T.);
#2952=ORIENTED_EDGE('',*,*,#2328,.T.);
#2953=ORIENTED_EDGE('',*,*,#2331,.T.);
#2954=ORIENTED_EDGE('',*,*,#2352,.T.);
#2955=ORIENTED_EDGE('',*,*,#2348,.T.);
#2956=ORIENTED_EDGE('',*,*,#2278,.T.);
#2957=ORIENTED_EDGE('',*,*,#2282,.T.);
#2958=ORIENTED_EDGE('',*,*,#2285,.T.);
#2959=ORIENTED_EDGE('',*,*,#2288,.T.);
#2960=ORIENTED_EDGE('',*,*,#2291,.T.);
#2961=ORIENTED_EDGE('',*,*,#2294,.T.);
#2962=ORIENTED_EDGE('',*,*,#2297,.T.);
#2963=ORIENTED_EDGE('',*,*,#2300,.T.);
#2964=ORIENTED_EDGE('',*,*,#2303,.T.);
#2965=ORIENTED_EDGE('',*,*,#2347,.T.);
#2966=ORIENTED_EDGE('',*,*,#2343,.T.);
#2967=ORIENTED_EDGE('',*,*,#2250,.T.);
#2968=ORIENTED_EDGE('',*,*,#2254,.T.);
#2969=ORIENTED_EDGE('',*,*,#2257,.T.);
#2970=ORIENTED_EDGE('',*,*,#2260,.T.);
#2971=ORIENTED_EDGE('',*,*,#2263,.T.);
#2972=ORIENTED_EDGE('',*,*,#2266,.T.);
#2973=ORIENTED_EDGE('',*,*,#2269,.T.);
#2974=ORIENTED_EDGE('',*,*,#2272,.T.);
#2975=ORIENTED_EDGE('',*,*,#2275,.T.);
#2976=ORIENTED_EDGE('',*,*,#2342,.T.);
#2977=ORIENTED_EDGE('',*,*,#2338,.T.);
#2978=ORIENTED_EDGE('',*,*,#2334,.T.);
#2979=ORIENTED_EDGE('',*,*,#2220,.T.);
#2980=ORIENTED_EDGE('',*,*,#2340,.F.);
#2981=ORIENTED_EDGE('',*,*,#2341,.F.);
#2982=ORIENTED_EDGE('',*,*,#2273,.T.);
#2983=ORIENTED_EDGE('',*,*,#2270,.T.);
#2984=ORIENTED_EDGE('',*,*,#2267,.T.);
#2985=ORIENTED_EDGE('',*,*,#2264,.T.);
#2986=ORIENTED_EDGE('',*,*,#2261,.T.);
#2987=ORIENTED_EDGE('',*,*,#2258,.T.);
#2988=ORIENTED_EDGE('',*,*,#2255,.T.);
#2989=ORIENTED_EDGE('',*,*,#2252,.T.);
#2990=ORIENTED_EDGE('',*,*,#2248,.T.);
#2991=ORIENTED_EDGE('',*,*,#2345,.F.);
#2992=ORIENTED_EDGE('',*,*,#2346,.F.);
#2993=ORIENTED_EDGE('',*,*,#2301,.T.);
#2994=ORIENTED_EDGE('',*,*,#2298,.T.);
#2995=ORIENTED_EDGE('',*,*,#2295,.T.);
#2996=ORIENTED_EDGE('',*,*,#2292,.T.);
#2997=ORIENTED_EDGE('',*,*,#2289,.T.);
#2998=ORIENTED_EDGE('',*,*,#2286,.T.);
#2999=ORIENTED_EDGE('',*,*,#2283,.T.);
#3000=ORIENTED_EDGE('',*,*,#2280,.T.);
#3001=ORIENTED_EDGE('',*,*,#2276,.T.);
#3002=ORIENTED_EDGE('',*,*,#2350,.F.);
#3003=ORIENTED_EDGE('',*,*,#2351,.F.);
#3004=ORIENTED_EDGE('',*,*,#2329,.T.);
#3005=ORIENTED_EDGE('',*,*,#2326,.T.);
#3006=ORIENTED_EDGE('',*,*,#2323,.T.);
#3007=ORIENTED_EDGE('',*,*,#2320,.T.);
#3008=ORIENTED_EDGE('',*,*,#2317,.T.);
#3009=ORIENTED_EDGE('',*,*,#2314,.T.);
#3010=ORIENTED_EDGE('',*,*,#2311,.T.);
#3011=ORIENTED_EDGE('',*,*,#2308,.T.);
#3012=ORIENTED_EDGE('',*,*,#2304,.T.);
#3013=ORIENTED_EDGE('',*,*,#2354,.F.);
#3014=ORIENTED_EDGE('',*,*,#2335,.F.);
#3015=ORIENTED_EDGE('',*,*,#2245,.T.);
#3016=ORIENTED_EDGE('',*,*,#2242,.T.);
#3017=ORIENTED_EDGE('',*,*,#2239,.T.);
#3018=ORIENTED_EDGE('',*,*,#2236,.T.);
#3019=ORIENTED_EDGE('',*,*,#2233,.T.);
#3020=ORIENTED_EDGE('',*,*,#2230,.T.);
#3021=ORIENTED_EDGE('',*,*,#2227,.T.);
#3022=ORIENTED_EDGE('',*,*,#2224,.T.);
#3023=ORIENTED_EDGE('',*,*,#2332,.T.);
#3822=PLANE('',#4429);
#3823=PLANE('',#4430);
#3824=PLANE('',#4431);
#3825=PLANE('',#4432);
#3826=PLANE('',#4433);
#3827=PLANE('',#4434);
#3828=PLANE('',#4435);
#3829=PLANE('',#4436);
#3830=PLANE('',#4437);
#3831=PLANE('',#4438);
#3832=PLANE('',#4439);
#3833=PLANE('',#4440);
#3834=PLANE('',#4441);
#3835=PLANE('',#4442);
#3836=PLANE('',#4443);
#3837=PLANE('',#4444);
#3838=PLANE('',#4445);
#3839=PLANE('',#4446);
#3840=PLANE('',#4447);
#3841=PLANE('',#4448);
#3842=PLANE('',#4449);
#3843=PLANE('',#4450);
#3844=PLANE('',#4451);
#3845=PLANE('',#4452);
#3846=PLANE('',#4453);
#3847=PLANE('',#4454);
#3848=PLANE('',#4455);
#3849=PLANE('',#4456);
#3850=PLANE('',#4457);
#3851=PLANE('',#4458);
#3852=PLANE('',#4459);
#3853=PLANE('',#4460);
#3854=PLANE('',#4461);
#3855=PLANE('',#4462);
#3856=PLANE('',#4463);
#3857=PLANE('',#4464);
#3858=PLANE('',#4468);
#3859=PLANE('',#4469);
#3860=PLANE('',#4470);
#3861=PLANE('',#4471);
#3862=PLANE('',#4472);
#3863=PLANE('',#4473);
#3864=PLANE('',#4474);
#3865=PLANE('',#4475);
#3866=PLANE('',#4476);
#3867=PLANE('',#4477);
#3967=ADVANCED_FACE('',(#652),#3822,.F.);
#3968=ADVANCED_FACE('',(#653),#3823,.F.);
#3969=ADVANCED_FACE('',(#654),#3824,.F.);
#3970=ADVANCED_FACE('',(#655),#3825,.F.);
#3971=ADVANCED_FACE('',(#656),#3826,.F.);
#3972=ADVANCED_FACE('',(#657),#3827,.F.);
#3973=ADVANCED_FACE('',(#658),#3828,.F.);
#3974=ADVANCED_FACE('',(#659),#3829,.F.);
#3975=ADVANCED_FACE('',(#660),#3830,.F.);
#3976=ADVANCED_FACE('',(#661),#3831,.F.);
#3977=ADVANCED_FACE('',(#662),#3832,.F.);
#3978=ADVANCED_FACE('',(#663),#3833,.F.);
#3979=ADVANCED_FACE('',(#664),#3834,.F.);
#3980=ADVANCED_FACE('',(#665),#3835,.F.);
#3981=ADVANCED_FACE('',(#666),#3836,.F.);
#3982=ADVANCED_FACE('',(#667),#3837,.F.);
#3983=ADVANCED_FACE('',(#668),#3838,.F.);
#3984=ADVANCED_FACE('',(#669),#3839,.F.);
#3985=ADVANCED_FACE('',(#670),#3840,.F.);
#3986=ADVANCED_FACE('',(#671),#3841,.F.);
#3987=ADVANCED_FACE('',(#672),#3842,.F.);
#3988=ADVANCED_FACE('',(#673),#3843,.F.);
#3989=ADVANCED_FACE('',(#674),#3844,.F.);
#3990=ADVANCED_FACE('',(#675),#3845,.F.);
#3991=ADVANCED_FACE('',(#676),#3846,.F.);
#3992=ADVANCED_FACE('',(#677),#3847,.F.);
#3993=ADVANCED_FACE('',(#678),#3848,.F.);
#3994=ADVANCED_FACE('',(#679),#3849,.F.);
#3995=ADVANCED_FACE('',(#680),#3850,.F.);
#3996=ADVANCED_FACE('',(#681),#3851,.F.);
#3997=ADVANCED_FACE('',(#682),#3852,.F.);
#3998=ADVANCED_FACE('',(#683),#3853,.F.);
#3999=ADVANCED_FACE('',(#684),#3854,.F.);
#4000=ADVANCED_FACE('',(#685),#3855,.F.);
#4001=ADVANCED_FACE('',(#686),#3856,.F.);
#4002=ADVANCED_FACE('',(#687),#3857,.F.);
#4003=ADVANCED_FACE('',(#688),#594,.F.);
#4004=ADVANCED_FACE('',(#689),#3858,.T.);
#4005=ADVANCED_FACE('',(#690),#3859,.T.);
#4006=ADVANCED_FACE('',(#691),#3860,.T.);
#4007=ADVANCED_FACE('',(#692),#3861,.T.);
#4008=ADVANCED_FACE('',(#693),#3862,.T.);
#4009=ADVANCED_FACE('',(#694),#3863,.T.);
#4010=ADVANCED_FACE('',(#695),#3864,.T.);
#4011=ADVANCED_FACE('',(#696),#3865,.T.);
#4012=ADVANCED_FACE('',(#697,#362),#3866,.T.);
#4013=ADVANCED_FACE('',(#698,#363),#3867,.F.);
#4199=CLOSED_SHELL('',(#3967,#3968,#3969,#3970,#3971,#3972,#3973,#3974,
#3975,#3976,#3977,#3978,#3979,#3980,#3981,#3982,#3983,#3984,#3985,#3986,
#3987,#3988,#3989,#3990,#3991,#3992,#3993,#3994,#3995,#3996,#3997,#3998,
#3999,#4000,#4001,#4002,#4003,#4004,#4005,#4006,#4007,#4008,#4009,#4010,
#4011,#4012,#4013));
#4428=AXIS2_PLACEMENT_3D('',#6218,#4913,#4914);
#4429=AXIS2_PLACEMENT_3D('',#6219,#4915,#4916);
#4430=AXIS2_PLACEMENT_3D('',#6228,#4921,#4922);
#4431=AXIS2_PLACEMENT_3D('',#6234,#4926,#4927);
#4432=AXIS2_PLACEMENT_3D('',#6240,#4931,#4932);
#4433=AXIS2_PLACEMENT_3D('',#6246,#4936,#4937);
#4434=AXIS2_PLACEMENT_3D('',#6252,#4941,#4942);
#4435=AXIS2_PLACEMENT_3D('',#6258,#4946,#4947);
#4436=AXIS2_PLACEMENT_3D('',#6264,#4951,#4952);
#4437=AXIS2_PLACEMENT_3D('',#6270,#4956,#4957);
#4438=AXIS2_PLACEMENT_3D('',#6276,#4961,#4962);
#4439=AXIS2_PLACEMENT_3D('',#6285,#4967,#4968);
#4440=AXIS2_PLACEMENT_3D('',#6291,#4972,#4973);
#4441=AXIS2_PLACEMENT_3D('',#6297,#4977,#4978);
#4442=AXIS2_PLACEMENT_3D('',#6303,#4982,#4983);
#4443=AXIS2_PLACEMENT_3D('',#6309,#4987,#4988);
#4444=AXIS2_PLACEMENT_3D('',#6315,#4992,#4993);
#4445=AXIS2_PLACEMENT_3D('',#6321,#4997,#4998);
#4446=AXIS2_PLACEMENT_3D('',#6327,#5002,#5003);
#4447=AXIS2_PLACEMENT_3D('',#6333,#5007,#5008);
#4448=AXIS2_PLACEMENT_3D('',#6342,#5013,#5014);
#4449=AXIS2_PLACEMENT_3D('',#6348,#5018,#5019);
#4450=AXIS2_PLACEMENT_3D('',#6354,#5023,#5024);
#4451=AXIS2_PLACEMENT_3D('',#6360,#5028,#5029);
#4452=AXIS2_PLACEMENT_3D('',#6366,#5033,#5034);
#4453=AXIS2_PLACEMENT_3D('',#6372,#5038,#5039);
#4454=AXIS2_PLACEMENT_3D('',#6378,#5043,#5044);
#4455=AXIS2_PLACEMENT_3D('',#6384,#5048,#5049);
#4456=AXIS2_PLACEMENT_3D('',#6390,#5053,#5054);
#4457=AXIS2_PLACEMENT_3D('',#6399,#5059,#5060);
#4458=AXIS2_PLACEMENT_3D('',#6405,#5064,#5065);
#4459=AXIS2_PLACEMENT_3D('',#6411,#5069,#5070);
#4460=AXIS2_PLACEMENT_3D('',#6417,#5074,#5075);
#4461=AXIS2_PLACEMENT_3D('',#6423,#5079,#5080);
#4462=AXIS2_PLACEMENT_3D('',#6429,#5084,#5085);
#4463=AXIS2_PLACEMENT_3D('',#6435,#5089,#5090);
#4464=AXIS2_PLACEMENT_3D('',#6441,#5094,#5095);
#4465=AXIS2_PLACEMENT_3D('',#6447,#5099,#5100);
#4466=AXIS2_PLACEMENT_3D('',#6449,#5101,#5102);
#4467=AXIS2_PLACEMENT_3D('',#6452,#5104,#5105);
#4468=AXIS2_PLACEMENT_3D('',#6453,#5106,#5107);
#4469=AXIS2_PLACEMENT_3D('',#6459,#5111,#5112);
#4470=AXIS2_PLACEMENT_3D('',#6465,#5116,#5117);
#4471=AXIS2_PLACEMENT_3D('',#6468,#5120,#5121);
#4472=AXIS2_PLACEMENT_3D('',#6474,#5125,#5126);
#4473=AXIS2_PLACEMENT_3D('',#6477,#5129,#5130);
#4474=AXIS2_PLACEMENT_3D('',#6483,#5134,#5135);
#4475=AXIS2_PLACEMENT_3D('',#6486,#5138,#5139);
#4476=AXIS2_PLACEMENT_3D('',#6489,#5142,#5143);
#4477=AXIS2_PLACEMENT_3D('',#6490,#5144,#5145);
#4913=DIRECTION('axis',(0.,0.,1.));
#4914=DIRECTION('refdir',(1.,0.,0.));
#4915=DIRECTION('center_axis',(0.,0.,-1.));
#4916=DIRECTION('ref_axis',(0.,1.,0.));
#4917=DIRECTION('',(0.,1.,0.));
#4918=DIRECTION('',(1.,0.,0.));
#4919=DIRECTION('',(0.,-1.,0.));
#4920=DIRECTION('',(1.,0.,0.));
#4921=DIRECTION('center_axis',(0.,1.,-8.88178419700125E-16));
#4922=DIRECTION('ref_axis',(0.,8.88178419700125E-16,1.));
#4923=DIRECTION('',(0.,8.88178419700125E-16,1.));
#4924=DIRECTION('',(1.,0.,0.));
#4925=DIRECTION('',(0.,-8.88178419700125E-16,-1.));
#4926=DIRECTION('center_axis',(0.,-7.40148683083439E-16,-1.));
#4927=DIRECTION('ref_axis',(0.,1.,-7.40148683083439E-16));
#4928=DIRECTION('',(0.,1.,-7.40148683083439E-16));
#4929=DIRECTION('',(1.,0.,0.));
#4930=DIRECTION('',(0.,-1.,7.40148683083439E-16));
#4931=DIRECTION('center_axis',(0.,-0.707106781186547,-0.707106781186548));
#4932=DIRECTION('ref_axis',(0.,0.707106781186548,-0.707106781186547));
#4933=DIRECTION('',(0.,0.707106781186548,-0.707106781186547));
#4934=DIRECTION('',(1.,0.,0.));
#4935=DIRECTION('',(0.,-0.707106781186548,0.707106781186547));
#4936=DIRECTION('center_axis',(0.,-1.,2.77555756156289E-16));
#4937=DIRECTION('ref_axis',(0.,-2.77555756156289E-16,-1.));
#4938=DIRECTION('',(0.,-2.77555756156289E-16,-1.));
#4939=DIRECTION('',(1.,0.,0.));
#4940=DIRECTION('',(0.,2.77555756156289E-16,1.));
#4941=DIRECTION('center_axis',(0.,-0.707106781186547,0.707106781186548));
#4942=DIRECTION('ref_axis',(0.,-0.707106781186548,-0.707106781186547));
#4943=DIRECTION('',(0.,-0.707106781186548,-0.707106781186547));
#4944=DIRECTION('',(1.,0.,0.));
#4945=DIRECTION('',(0.,0.707106781186548,0.707106781186547));
#4946=DIRECTION('center_axis',(0.,7.40148683083438E-16,1.));
#4947=DIRECTION('ref_axis',(0.,-1.,7.40148683083438E-16));
#4948=DIRECTION('',(0.,-1.,7.40148683083438E-16));
#4949=DIRECTION('',(1.,0.,0.));
#4950=DIRECTION('',(0.,1.,-7.40148683083438E-16));
#4951=DIRECTION('center_axis',(0.,1.,-4.44089209850063E-16));
#4952=DIRECTION('ref_axis',(0.,4.44089209850063E-16,1.));
#4953=DIRECTION('',(0.,4.44089209850063E-16,1.));
#4954=DIRECTION('',(1.,0.,0.));
#4955=DIRECTION('',(0.,-4.44089209850063E-16,-1.));
#4956=DIRECTION('center_axis',(0.,2.41352831440251E-16,1.));
#4957=DIRECTION('ref_axis',(0.,-1.,2.41352831440251E-16));
#4958=DIRECTION('',(0.,-1.,2.41352831440251E-16));
#4959=DIRECTION('',(-1.,0.,0.));
#4960=DIRECTION('',(0.,1.,-2.41352831440251E-16));
#4961=DIRECTION('center_axis',(0.,-1.,2.41352831440251E-16));
#4962=DIRECTION('ref_axis',(0.,-2.41352831440251E-16,-1.));
#4963=DIRECTION('',(0.,-2.41352831440251E-16,-1.));
#4964=DIRECTION('',(1.,0.,0.));
#4965=DIRECTION('',(0.,2.41352831440251E-16,1.));
#4966=DIRECTION('',(1.,0.,0.));
#4967=DIRECTION('center_axis',(0.,0.,-1.));
#4968=DIRECTION('ref_axis',(0.,1.,0.));
#4969=DIRECTION('',(0.,1.,0.));
#4970=DIRECTION('',(1.,0.,0.));
#4971=DIRECTION('',(0.,-1.,0.));
#4972=DIRECTION('center_axis',(0.,-1.,0.));
#4973=DIRECTION('ref_axis',(0.,0.,-1.));
#4974=DIRECTION('',(0.,0.,-1.));
#4975=DIRECTION('',(1.,0.,0.));
#4976=DIRECTION('',(0.,0.,1.));
#4977=DIRECTION('center_axis',(0.,-0.707106781186547,0.707106781186548));
#4978=DIRECTION('ref_axis',(0.,-0.707106781186548,-0.707106781186547));
#4979=DIRECTION('',(0.,-0.707106781186548,-0.707106781186547));
#4980=DIRECTION('',(1.,0.,0.));
#4981=DIRECTION('',(0.,0.707106781186548,0.707106781186547));
#4982=DIRECTION('center_axis',(0.,0.,1.));
#4983=DIRECTION('ref_axis',(0.,-1.,0.));
#4984=DIRECTION('',(0.,-1.,0.));
#4985=DIRECTION('',(1.,0.,0.));
#4986=DIRECTION('',(0.,1.,0.));
#4987=DIRECTION('center_axis',(0.,0.707106781186548,0.707106781186547));
#4988=DIRECTION('ref_axis',(0.,-0.707106781186547,0.707106781186548));
#4989=DIRECTION('',(0.,-0.707106781186547,0.707106781186548));
#4990=DIRECTION('',(1.,0.,0.));
#4991=DIRECTION('',(0.,0.707106781186547,-0.707106781186548));
#4992=DIRECTION('center_axis',(0.,1.,0.));
#4993=DIRECTION('ref_axis',(0.,0.,1.));
#4994=DIRECTION('',(0.,0.,1.));
#4995=DIRECTION('',(1.,0.,0.));
#4996=DIRECTION('',(0.,0.,-1.));
#4997=DIRECTION('center_axis',(0.,0.,-1.));
#4998=DIRECTION('ref_axis',(0.,1.,0.));
#4999=DIRECTION('',(0.,1.,0.));
#5000=DIRECTION('',(1.,0.,0.));
#5001=DIRECTION('',(0.,-1.,0.));
#5002=DIRECTION('center_axis',(0.,1.,-2.41352831440251E-16));
#5003=DIRECTION('ref_axis',(0.,2.41352831440251E-16,1.));
#5004=DIRECTION('',(0.,2.41352831440251E-16,1.));
#5005=DIRECTION('',(-1.,0.,0.));
#5006=DIRECTION('',(0.,-2.41352831440251E-16,-1.));
#5007=DIRECTION('center_axis',(0.,0.,1.));
#5008=DIRECTION('ref_axis',(0.,-1.,0.));
#5009=DIRECTION('',(0.,-1.,0.));
#5010=DIRECTION('',(1.,0.,0.));
#5011=DIRECTION('',(0.,1.,0.));
#5012=DIRECTION('',(1.,0.,0.));
#5013=DIRECTION('center_axis',(0.,-1.,0.));
#5014=DIRECTION('ref_axis',(0.,0.,-1.));
#5015=DIRECTION('',(0.,0.,-1.));
#5016=DIRECTION('',(1.,0.,0.));
#5017=DIRECTION('',(0.,0.,1.));
#5018=DIRECTION('center_axis',(0.,0.,1.));
#5019=DIRECTION('ref_axis',(0.,-1.,0.));
#5020=DIRECTION('',(0.,-1.,0.));
#5021=DIRECTION('',(1.,0.,0.));
#5022=DIRECTION('',(0.,1.,0.));
#5023=DIRECTION('center_axis',(0.,0.707106781186548,0.707106781186548));
#5024=DIRECTION('ref_axis',(0.,-0.707106781186548,0.707106781186548));
#5025=DIRECTION('',(0.,-0.707106781186548,0.707106781186548));
#5026=DIRECTION('',(1.,0.,0.));
#5027=DIRECTION('',(0.,0.707106781186548,-0.707106781186548));
#5028=DIRECTION('center_axis',(0.,1.,0.));
#5029=DIRECTION('ref_axis',(0.,0.,1.));
#5030=DIRECTION('',(0.,0.,1.));
#5031=DIRECTION('',(1.,0.,0.));
#5032=DIRECTION('',(0.,0.,-1.));
#5033=DIRECTION('center_axis',(0.,0.707106781186548,-0.707106781186547));
#5034=DIRECTION('ref_axis',(0.,0.707106781186547,0.707106781186548));
#5035=DIRECTION('',(0.,0.707106781186547,0.707106781186548));
#5036=DIRECTION('',(1.,0.,0.));
#5037=DIRECTION('',(0.,-0.707106781186547,-0.707106781186548));
#5038=DIRECTION('center_axis',(0.,-7.40148683083438E-16,-1.));
#5039=DIRECTION('ref_axis',(0.,1.,-7.40148683083438E-16));
#5040=DIRECTION('',(0.,1.,-7.40148683083438E-16));
#5041=DIRECTION('',(1.,0.,0.));
#5042=DIRECTION('',(0.,-1.,7.40148683083438E-16));
#5043=DIRECTION('center_axis',(0.,-1.,0.));
#5044=DIRECTION('ref_axis',(0.,0.,-1.));
#5045=DIRECTION('',(0.,0.,-1.));
#5046=DIRECTION('',(1.,0.,0.));
#5047=DIRECTION('',(0.,0.,1.));
#5048=DIRECTION('center_axis',(0.,0.,-1.));
#5049=DIRECTION('ref_axis',(0.,1.,0.));
#5050=DIRECTION('',(0.,1.,0.));
#5051=DIRECTION('',(-1.,0.,0.));
#5052=DIRECTION('',(0.,-1.,0.));
#5053=DIRECTION('center_axis',(0.,1.,0.));
#5054=DIRECTION('ref_axis',(0.,0.,1.));
#5055=DIRECTION('',(0.,0.,1.));
#5056=DIRECTION('',(1.,0.,0.));
#5057=DIRECTION('',(0.,0.,-1.));
#5058=DIRECTION('',(1.,0.,0.));
#5059=DIRECTION('center_axis',(0.,0.,1.));
#5060=DIRECTION('ref_axis',(0.,-1.,0.));
#5061=DIRECTION('',(0.,-1.,0.));
#5062=DIRECTION('',(1.,0.,0.));
#5063=DIRECTION('',(0.,1.,0.));
#5064=DIRECTION('center_axis',(0.,1.,0.));
#5065=DIRECTION('ref_axis',(0.,0.,1.));
#5066=DIRECTION('',(0.,0.,1.));
#5067=DIRECTION('',(1.,0.,0.));
#5068=DIRECTION('',(0.,0.,-1.));
#5069=DIRECTION('center_axis',(0.,0.707106781186547,-0.707106781186548));
#5070=DIRECTION('ref_axis',(0.,0.707106781186548,0.707106781186547));
#5071=DIRECTION('',(0.,0.707106781186548,0.707106781186547));
#5072=DIRECTION('',(1.,0.,0.));
#5073=DIRECTION('',(0.,-0.707106781186548,-0.707106781186547));
#5074=DIRECTION('center_axis',(0.,0.,-1.));
#5075=DIRECTION('ref_axis',(0.,1.,0.));
#5076=DIRECTION('',(0.,1.,0.));
#5077=DIRECTION('',(1.,0.,0.));
#5078=DIRECTION('',(0.,-1.,0.));
#5079=DIRECTION('center_axis',(0.,-0.707106781186547,-0.707106781186548));
#5080=DIRECTION('ref_axis',(0.,0.707106781186548,-0.707106781186547));
#5081=DIRECTION('',(0.,0.707106781186548,-0.707106781186547));
#5082=DIRECTION('',(1.,0.,0.));
#5083=DIRECTION('',(0.,-0.707106781186548,0.707106781186547));
#5084=DIRECTION('center_axis',(0.,-1.,0.));
#5085=DIRECTION('ref_axis',(0.,0.,-1.));
#5086=DIRECTION('',(0.,0.,-1.));
#5087=DIRECTION('',(1.,0.,0.));
#5088=DIRECTION('',(0.,0.,1.));
#5089=DIRECTION('center_axis',(0.,0.,1.));
#5090=DIRECTION('ref_axis',(0.,-1.,0.));
#5091=DIRECTION('',(0.,-1.,0.));
#5092=DIRECTION('',(1.,0.,0.));
#5093=DIRECTION('',(0.,1.,0.));
#5094=DIRECTION('center_axis',(0.,-1.,0.));
#5095=DIRECTION('ref_axis',(0.,0.,-1.));
#5096=DIRECTION('',(0.,0.,-1.));
#5097=DIRECTION('',(-1.,0.,0.));
#5098=DIRECTION('',(0.,0.,1.));
#5099=DIRECTION('center_axis',(1.,0.,0.));
#5100=DIRECTION('ref_axis',(0.,0.,-1.));
#5101=DIRECTION('center_axis',(1.,0.,0.));
#5102=DIRECTION('ref_axis',(0.,0.,-1.));
#5103=DIRECTION('',(1.,0.,0.));
#5104=DIRECTION('center_axis',(-1.,0.,0.));
#5105=DIRECTION('ref_axis',(0.,0.,-1.));
#5106=DIRECTION('center_axis',(0.,1.,0.));
#5107=DIRECTION('ref_axis',(0.,0.,1.));
#5108=DIRECTION('',(0.,0.,1.));
#5109=DIRECTION('',(1.,0.,0.));
#5110=DIRECTION('',(0.,0.,1.));
#5111=DIRECTION('center_axis',(0.,1.,0.));
#5112=DIRECTION('ref_axis',(0.,0.,1.));
#5113=DIRECTION('',(0.,0.,1.));
#5114=DIRECTION('',(1.,0.,0.));
#5115=DIRECTION('',(0.,0.,1.));
#5116=DIRECTION('center_axis',(0.,0.,-1.));
#5117=DIRECTION('ref_axis',(0.,1.,0.));
#5118=DIRECTION('',(0.,1.,0.));
#5119=DIRECTION('',(0.,1.,0.));
#5120=DIRECTION('center_axis',(0.,0.,-1.));
#5121=DIRECTION('ref_axis',(0.,1.,0.));
#5122=DIRECTION('',(0.,1.,0.));
#5123=DIRECTION('',(1.,0.,0.));
#5124=DIRECTION('',(0.,1.,0.));
#5125=DIRECTION('center_axis',(0.,-1.,0.));
#5126=DIRECTION('ref_axis',(0.,0.,-1.));
#5127=DIRECTION('',(0.,0.,-1.));
#5128=DIRECTION('',(0.,0.,-1.));
#5129=DIRECTION('center_axis',(0.,-1.,0.));
#5130=DIRECTION('ref_axis',(0.,0.,-1.));
#5131=DIRECTION('',(0.,0.,-1.));
#5132=DIRECTION('',(1.,0.,0.));
#5133=DIRECTION('',(0.,0.,-1.));
#5134=DIRECTION('center_axis',(0.,0.,1.));
#5135=DIRECTION('ref_axis',(0.,-1.,0.));
#5136=DIRECTION('',(0.,-1.,0.));
#5137=DIRECTION('',(0.,-1.,0.));
#5138=DIRECTION('center_axis',(0.,0.,1.));
#5139=DIRECTION('ref_axis',(0.,-1.,0.));
#5140=DIRECTION('',(0.,-1.,0.));
#5141=DIRECTION('',(0.,-1.,0.));
#5142=DIRECTION('center_axis',(1.,0.,0.));
#5143=DIRECTION('ref_axis',(0.,0.,-1.));
#5144=DIRECTION('center_axis',(1.,0.,0.));
#5145=DIRECTION('ref_axis',(0.,0.,-1.));
#6218=CARTESIAN_POINT('',(0.,0.,0.));
#6219=CARTESIAN_POINT('Origin',(-0.1,0.82,-0.3));
#6220=CARTESIAN_POINT('',(0.,0.82,-0.3));
#6221=CARTESIAN_POINT('',(0.,1.,-0.3));
#6222=CARTESIAN_POINT('',(0.,0.41,-0.3));
#6223=CARTESIAN_POINT('',(30.,0.82,-0.3));
#6224=CARTESIAN_POINT('',(-0.1,0.82,-0.3));
#6225=CARTESIAN_POINT('',(30.,1.,-0.3));
#6226=CARTESIAN_POINT('',(30.,0.41,-0.3));
#6227=CARTESIAN_POINT('',(-0.05,1.,-0.3));
#6228=CARTESIAN_POINT('Origin',(-0.1,0.82,-0.55));
#6229=CARTESIAN_POINT('',(0.,0.82,-0.55));
#6230=CARTESIAN_POINT('',(0.,0.82,-0.275));
#6231=CARTESIAN_POINT('',(30.,0.82,-0.55));
#6232=CARTESIAN_POINT('',(-0.1,0.82,-0.55));
#6233=CARTESIAN_POINT('',(30.,0.82,-0.275));
#6234=CARTESIAN_POINT('Origin',(-0.1,0.67,-0.55));
#6235=CARTESIAN_POINT('',(0.,0.67,-0.55));
#6236=CARTESIAN_POINT('',(0.,0.335,-0.55));
#6237=CARTESIAN_POINT('',(30.,0.67,-0.55));
#6238=CARTESIAN_POINT('',(-0.1,0.67,-0.55));
#6239=CARTESIAN_POINT('',(30.,0.335,-0.55));
#6240=CARTESIAN_POINT('Origin',(-0.1,0.42,-0.3));
#6241=CARTESIAN_POINT('',(0.,0.42,-0.3));
#6242=CARTESIAN_POINT('',(0.,0.24,-0.12));
#6243=CARTESIAN_POINT('',(30.,0.42,-0.3));
#6244=CARTESIAN_POINT('',(-0.1,0.42,-0.3));
#6245=CARTESIAN_POINT('',(30.,0.24,-0.12));
#6246=CARTESIAN_POINT('Origin',(-0.1,0.42,0.3));
#6247=CARTESIAN_POINT('',(0.,0.42,0.3));
#6248=CARTESIAN_POINT('',(0.,0.42,0.15));
#6249=CARTESIAN_POINT('',(30.,0.42,0.3));
#6250=CARTESIAN_POINT('',(-0.1,0.42,0.3));
#6251=CARTESIAN_POINT('',(30.,0.42,0.15));
#6252=CARTESIAN_POINT('Origin',(-0.1,0.67,0.55));
#6253=CARTESIAN_POINT('',(0.,0.67,0.55));
#6254=CARTESIAN_POINT('',(6.93889390390723E-18,0.365,0.245));
#6255=CARTESIAN_POINT('',(30.,0.67,0.55));
#6256=CARTESIAN_POINT('',(-0.1,0.67,0.55));
#6257=CARTESIAN_POINT('',(30.,0.365,0.245));
#6258=CARTESIAN_POINT('Origin',(-0.1,0.82,0.55));
#6259=CARTESIAN_POINT('',(0.,0.82,0.55));
#6260=CARTESIAN_POINT('',(0.,0.41,0.55));
#6261=CARTESIAN_POINT('',(30.,0.82,0.55));
#6262=CARTESIAN_POINT('',(-0.1,0.82,0.55));
#6263=CARTESIAN_POINT('',(30.,0.41,0.55));
#6264=CARTESIAN_POINT('Origin',(-0.1,0.82,0.3));
#6265=CARTESIAN_POINT('',(0.,0.82,0.3));
#6266=CARTESIAN_POINT('',(0.,0.82,0.15));
#6267=CARTESIAN_POINT('',(30.,0.82,0.3));
#6268=CARTESIAN_POINT('',(-0.1,0.82,0.3));
#6269=CARTESIAN_POINT('',(30.,0.82,0.15));
#6270=CARTESIAN_POINT('Origin',(-0.1,1.05,0.3));
#6271=CARTESIAN_POINT('',(0.,1.,0.3));
#6272=CARTESIAN_POINT('',(0.,0.525,0.3));
#6273=CARTESIAN_POINT('',(30.,1.,0.3));
#6274=CARTESIAN_POINT('',(-0.05,1.,0.3));
#6275=CARTESIAN_POINT('',(30.,0.525,0.3));
#6276=CARTESIAN_POINT('Origin',(-0.1,-0.3,-0.82));
#6277=CARTESIAN_POINT('',(0.,-0.3,-0.82));
#6278=CARTESIAN_POINT('',(0.,-0.3,-1.));
#6279=CARTESIAN_POINT('',(0.,-0.3,-0.41));
#6280=CARTESIAN_POINT('',(30.,-0.3,-0.82));
#6281=CARTESIAN_POINT('',(-0.1,-0.3,-0.82));
#6282=CARTESIAN_POINT('',(30.,-0.3,-1.));
#6283=CARTESIAN_POINT('',(30.,-0.3,-0.41));
#6284=CARTESIAN_POINT('',(-0.05,-0.3,-1.));
#6285=CARTESIAN_POINT('Origin',(-0.1,-0.55,-0.82));
#6286=CARTESIAN_POINT('',(0.,-0.55,-0.82));
#6287=CARTESIAN_POINT('',(0.,-0.275,-0.82));
#6288=CARTESIAN_POINT('',(30.,-0.55,-0.82));
#6289=CARTESIAN_POINT('',(-0.1,-0.55,-0.82));
#6290=CARTESIAN_POINT('',(30.,-0.275,-0.82));
#6291=CARTESIAN_POINT('Origin',(-0.1,-0.55,-0.67));
#6292=CARTESIAN_POINT('',(0.,-0.55,-0.67));
#6293=CARTESIAN_POINT('',(0.,-0.55,-0.335));
#6294=CARTESIAN_POINT('',(30.,-0.55,-0.67));
#6295=CARTESIAN_POINT('',(-0.1,-0.55,-0.67));
#6296=CARTESIAN_POINT('',(30.,-0.55,-0.335));
#6297=CARTESIAN_POINT('Origin',(-0.1,-0.3,-0.42));
#6298=CARTESIAN_POINT('',(0.,-0.3,-0.42));
#6299=CARTESIAN_POINT('',(0.,-0.12,-0.24));
#6300=CARTESIAN_POINT('',(30.,-0.3,-0.42));
#6301=CARTESIAN_POINT('',(-0.1,-0.3,-0.42));
#6302=CARTESIAN_POINT('',(30.,-0.12,-0.24));
#6303=CARTESIAN_POINT('Origin',(-0.1,0.3,-0.42));
#6304=CARTESIAN_POINT('',(0.,0.3,-0.42));
#6305=CARTESIAN_POINT('',(0.,0.15,-0.42));
#6306=CARTESIAN_POINT('',(30.,0.3,-0.42));
#6307=CARTESIAN_POINT('',(-0.1,0.3,-0.42));
#6308=CARTESIAN_POINT('',(30.,0.15,-0.42));
#6309=CARTESIAN_POINT('Origin',(-0.1,0.55,-0.67));
#6310=CARTESIAN_POINT('',(0.,0.55,-0.67));
#6311=CARTESIAN_POINT('',(0.,0.245,-0.365));
#6312=CARTESIAN_POINT('',(30.,0.55,-0.67));
#6313=CARTESIAN_POINT('',(-0.1,0.55,-0.67));
#6314=CARTESIAN_POINT('',(30.,0.245,-0.365));
#6315=CARTESIAN_POINT('Origin',(-0.1,0.55,-0.82));
#6316=CARTESIAN_POINT('',(0.,0.55,-0.82));
#6317=CARTESIAN_POINT('',(0.,0.55,-0.41));
#6318=CARTESIAN_POINT('',(30.,0.55,-0.82));
#6319=CARTESIAN_POINT('',(-0.1,0.55,-0.82));
#6320=CARTESIAN_POINT('',(30.,0.55,-0.41));
#6321=CARTESIAN_POINT('Origin',(-0.1,0.3,-0.82));
#6322=CARTESIAN_POINT('',(0.,0.3,-0.82));
#6323=CARTESIAN_POINT('',(0.,0.15,-0.82));
#6324=CARTESIAN_POINT('',(30.,0.3,-0.82));
#6325=CARTESIAN_POINT('',(-0.1,0.3,-0.82));
#6326=CARTESIAN_POINT('',(30.,0.15,-0.82));
#6327=CARTESIAN_POINT('Origin',(-0.1,0.3,-1.05));
#6328=CARTESIAN_POINT('',(0.,0.3,-1.));
#6329=CARTESIAN_POINT('',(0.,0.3,-0.525));
#6330=CARTESIAN_POINT('',(30.,0.3,-1.));
#6331=CARTESIAN_POINT('',(-0.05,0.3,-1.));
#6332=CARTESIAN_POINT('',(30.,0.3,-0.525));
#6333=CARTESIAN_POINT('Origin',(-0.1,-0.82,0.3));
#6334=CARTESIAN_POINT('',(0.,-0.82,0.3));
#6335=CARTESIAN_POINT('',(0.,-1.,0.3));
#6336=CARTESIAN_POINT('',(0.,-0.41,0.3));
#6337=CARTESIAN_POINT('',(30.,-0.82,0.3));
#6338=CARTESIAN_POINT('',(-0.1,-0.82,0.3));
#6339=CARTESIAN_POINT('',(30.,-1.,0.3));
#6340=CARTESIAN_POINT('',(30.,-0.41,0.3));
#6341=CARTESIAN_POINT('',(-0.05,-1.,0.3));
#6342=CARTESIAN_POINT('Origin',(-0.1,-0.82,0.55));
#6343=CARTESIAN_POINT('',(0.,-0.82,0.55));
#6344=CARTESIAN_POINT('',(0.,-0.82,0.275));
#6345=CARTESIAN_POINT('',(30.,-0.82,0.55));
#6346=CARTESIAN_POINT('',(-0.1,-0.82,0.55));
#6347=CARTESIAN_POINT('',(30.,-0.82,0.275));
#6348=CARTESIAN_POINT('Origin',(-0.1,-0.67,0.55));
#6349=CARTESIAN_POINT('',(0.,-0.67,0.55));
#6350=CARTESIAN_POINT('',(0.,-0.335,0.55));
#6351=CARTESIAN_POINT('',(30.,-0.67,0.55));
#6352=CARTESIAN_POINT('',(-0.1,-0.67,0.55));
#6353=CARTESIAN_POINT('',(30.,-0.335,0.55));
#6354=CARTESIAN_POINT('Origin',(-0.1,-0.42,0.3));
#6355=CARTESIAN_POINT('',(0.,-0.42,0.3));
#6356=CARTESIAN_POINT('',(-6.93889390390723E-18,-0.24,0.12));
#6357=CARTESIAN_POINT('',(30.,-0.42,0.3));
#6358=CARTESIAN_POINT('',(-0.1,-0.42,0.3));
#6359=CARTESIAN_POINT('',(30.,-0.24,0.12));
#6360=CARTESIAN_POINT('Origin',(-0.1,-0.42,-0.3));
#6361=CARTESIAN_POINT('',(0.,-0.42,-0.3));
#6362=CARTESIAN_POINT('',(0.,-0.42,-0.15));
#6363=CARTESIAN_POINT('',(30.,-0.42,-0.3));
#6364=CARTESIAN_POINT('',(-0.1,-0.42,-0.3));
#6365=CARTESIAN_POINT('',(30.,-0.42,-0.15));
#6366=CARTESIAN_POINT('Origin',(-0.1,-0.67,-0.55));
#6367=CARTESIAN_POINT('',(0.,-0.67,-0.55));
#6368=CARTESIAN_POINT('',(0.,-0.365,-0.245));
#6369=CARTESIAN_POINT('',(30.,-0.67,-0.55));
#6370=CARTESIAN_POINT('',(-0.1,-0.67,-0.55));
#6371=CARTESIAN_POINT('',(30.,-0.365,-0.245));
#6372=CARTESIAN_POINT('Origin',(-0.1,-0.82,-0.55));
#6373=CARTESIAN_POINT('',(0.,-0.82,-0.55));
#6374=CARTESIAN_POINT('',(0.,-0.41,-0.55));
#6375=CARTESIAN_POINT('',(30.,-0.82,-0.55));
#6376=CARTESIAN_POINT('',(-0.1,-0.82,-0.55));
#6377=CARTESIAN_POINT('',(30.,-0.41,-0.55));
#6378=CARTESIAN_POINT('Origin',(-0.1,-0.82,-0.3));
#6379=CARTESIAN_POINT('',(0.,-0.82,-0.3));
#6380=CARTESIAN_POINT('',(0.,-0.82,-0.15));
#6381=CARTESIAN_POINT('',(30.,-0.82,-0.3));
#6382=CARTESIAN_POINT('',(-0.1,-0.82,-0.3));
#6383=CARTESIAN_POINT('',(30.,-0.82,-0.15));
#6384=CARTESIAN_POINT('Origin',(-0.1,-1.05,-0.3));
#6385=CARTESIAN_POINT('',(0.,-1.,-0.3));
#6386=CARTESIAN_POINT('',(0.,-0.525,-0.3));
#6387=CARTESIAN_POINT('',(30.,-1.,-0.3));
#6388=CARTESIAN_POINT('',(-0.05,-1.,-0.3));
#6389=CARTESIAN_POINT('',(30.,-0.525,-0.3));
#6390=CARTESIAN_POINT('Origin',(-0.1,0.3,0.82));
#6391=CARTESIAN_POINT('',(0.,0.3,0.82));
#6392=CARTESIAN_POINT('',(0.,0.3,1.));
#6393=CARTESIAN_POINT('',(0.,0.3,0.41));
#6394=CARTESIAN_POINT('',(30.,0.3,0.82));
#6395=CARTESIAN_POINT('',(-0.1,0.3,0.82));
#6396=CARTESIAN_POINT('',(30.,0.3,1.));
#6397=CARTESIAN_POINT('',(30.,0.3,0.41));
#6398=CARTESIAN_POINT('',(-0.05,0.3,1.));
#6399=CARTESIAN_POINT('Origin',(-0.1,0.55,0.82));
#6400=CARTESIAN_POINT('',(0.,0.55,0.82));
#6401=CARTESIAN_POINT('',(0.,0.275,0.82));
#6402=CARTESIAN_POINT('',(30.,0.55,0.82));
#6403=CARTESIAN_POINT('',(-0.1,0.55,0.82));
#6404=CARTESIAN_POINT('',(30.,0.275,0.82));
#6405=CARTESIAN_POINT('Origin',(-0.1,0.55,0.67));
#6406=CARTESIAN_POINT('',(0.,0.55,0.67));
#6407=CARTESIAN_POINT('',(0.,0.55,0.335));
#6408=CARTESIAN_POINT('',(30.,0.55,0.67));
#6409=CARTESIAN_POINT('',(-0.1,0.55,0.67));
#6410=CARTESIAN_POINT('',(30.,0.55,0.335));
#6411=CARTESIAN_POINT('Origin',(-0.1,0.3,0.42));
#6412=CARTESIAN_POINT('',(0.,0.3,0.42));
#6413=CARTESIAN_POINT('',(6.93889390390723E-18,0.12,0.24));
#6414=CARTESIAN_POINT('',(30.,0.3,0.42));
#6415=CARTESIAN_POINT('',(-0.1,0.3,0.42));
#6416=CARTESIAN_POINT('',(30.,0.12,0.24));
#6417=CARTESIAN_POINT('Origin',(-0.1,-0.3,0.42));
#6418=CARTESIAN_POINT('',(0.,-0.3,0.42));
#6419=CARTESIAN_POINT('',(0.,-0.15,0.42));
#6420=CARTESIAN_POINT('',(30.,-0.3,0.42));
#6421=CARTESIAN_POINT('',(-0.1,-0.3,0.42));
#6422=CARTESIAN_POINT('',(30.,-0.15,0.42));
#6423=CARTESIAN_POINT('Origin',(-0.1,-0.55,0.67));
#6424=CARTESIAN_POINT('',(0.,-0.55,0.67));
#6425=CARTESIAN_POINT('',(6.93889390390723E-18,-0.245,0.365));
#6426=CARTESIAN_POINT('',(30.,-0.55,0.67));
#6427=CARTESIAN_POINT('',(-0.1,-0.55,0.67));
#6428=CARTESIAN_POINT('',(30.,-0.245,0.365));
#6429=CARTESIAN_POINT('Origin',(-0.1,-0.55,0.82));
#6430=CARTESIAN_POINT('',(0.,-0.55,0.82));
#6431=CARTESIAN_POINT('',(0.,-0.55,0.41));
#6432=CARTESIAN_POINT('',(30.,-0.55,0.82));
#6433=CARTESIAN_POINT('',(-0.1,-0.55,0.82));
#6434=CARTESIAN_POINT('',(30.,-0.55,0.41));
#6435=CARTESIAN_POINT('Origin',(-0.1,-0.3,0.82));
#6436=CARTESIAN_POINT('',(0.,-0.3,0.82));
#6437=CARTESIAN_POINT('',(0.,-0.15,0.82));
#6438=CARTESIAN_POINT('',(30.,-0.3,0.82));
#6439=CARTESIAN_POINT('',(-0.1,-0.3,0.82));
#6440=CARTESIAN_POINT('',(30.,-0.15,0.82));
#6441=CARTESIAN_POINT('Origin',(-0.1,-0.3,1.05));
#6442=CARTESIAN_POINT('',(0.,-0.3,1.));
#6443=CARTESIAN_POINT('',(0.,-0.3,0.525));
#6444=CARTESIAN_POINT('',(30.,-0.3,1.));
#6445=CARTESIAN_POINT('',(-0.05,-0.3,1.));
#6446=CARTESIAN_POINT('',(30.,-0.3,0.525));
#6447=CARTESIAN_POINT('Origin',(-0.1,0.,0.));
#6448=CARTESIAN_POINT('',(0.,-2.57175827820944E-17,0.21));
#6449=CARTESIAN_POINT('Origin',(0.,0.,0.));
#6450=CARTESIAN_POINT('',(30.,2.57175827820944E-17,0.21));
#6451=CARTESIAN_POINT('',(-0.1,-2.57175827820944E-17,0.21));
#6452=CARTESIAN_POINT('Origin',(30.,0.,0.));
#6453=CARTESIAN_POINT('Origin',(0.,1.,-1.));
#6454=CARTESIAN_POINT('',(0.,1.,1.));
#6455=CARTESIAN_POINT('',(0.,1.,-1.));
#6456=CARTESIAN_POINT('',(30.,1.,1.));
#6457=CARTESIAN_POINT('',(0.,1.,1.));
#6458=CARTESIAN_POINT('',(30.,1.,-1.));
#6459=CARTESIAN_POINT('Origin',(0.,1.,-1.));
#6460=CARTESIAN_POINT('',(30.,1.,-1.));
#6461=CARTESIAN_POINT('',(30.,1.,-1.));
#6462=CARTESIAN_POINT('',(0.,1.,-1.));
#6463=CARTESIAN_POINT('',(0.,1.,-1.));
#6464=CARTESIAN_POINT('',(0.,1.,-1.));
#6465=CARTESIAN_POINT('Origin',(0.,-1.,-1.));
#6466=CARTESIAN_POINT('',(0.,-1.,-1.));
#6467=CARTESIAN_POINT('',(30.,-1.,-1.));
#6468=CARTESIAN_POINT('Origin',(0.,-1.,-1.));
#6469=CARTESIAN_POINT('',(30.,-1.,-1.));
#6470=CARTESIAN_POINT('',(30.,-1.,-1.));
#6471=CARTESIAN_POINT('',(0.,-1.,-1.));
#6472=CARTESIAN_POINT('',(0.,-1.,-1.));
#6473=CARTESIAN_POINT('',(0.,-1.,-1.));
#6474=CARTESIAN_POINT('Origin',(0.,-1.,1.));
#6475=CARTESIAN_POINT('',(0.,-1.,1.));
#6476=CARTESIAN_POINT('',(30.,-1.,1.));
#6477=CARTESIAN_POINT('Origin',(0.,-1.,1.));
#6478=CARTESIAN_POINT('',(30.,-1.,1.));
#6479=CARTESIAN_POINT('',(30.,-1.,1.));
#6480=CARTESIAN_POINT('',(0.,-1.,1.));
#6481=CARTESIAN_POINT('',(0.,-1.,1.));
#6482=CARTESIAN_POINT('',(0.,-1.,1.));
#6483=CARTESIAN_POINT('Origin',(0.,1.,1.));
#6484=CARTESIAN_POINT('',(0.,1.,1.));
#6485=CARTESIAN_POINT('',(30.,1.,1.));
#6486=CARTESIAN_POINT('Origin',(0.,1.,1.));
#6487=CARTESIAN_POINT('',(30.,1.,1.));
#6488=CARTESIAN_POINT('',(0.,1.,1.));
#6489=CARTESIAN_POINT('Origin',(30.,0.,0.));
#6490=CARTESIAN_POINT('Origin',(0.,0.,0.));
#7761=UNCERTAINTY_MEASURE_WITH_UNIT(LENGTH_MEASURE(0.001),#7807,
'DISTANCE_ACCURACY_VALUE',
'Maximum model space distance between geometric entities at asserted c
onnectivities');
#7782=UNCERTAINTY_MEASURE_WITH_UNIT(LENGTH_MEASURE(0.001),#7807,
'DISTANCE_ACCURACY_VALUE',
'Maximum model space distance between geometric entities at asserted c
onnectivities');
#7785=(
GEOMETRIC_REPRESENTATION_CONTEXT(3)
GLOBAL_UNCERTAINTY_ASSIGNED_CONTEXT((#7761))
GLOBAL_UNIT_ASSIGNED_CONTEXT((#7807,#7809,#7810))
REPRESENTATION_CONTEXT('','3D')
);
#7806=(
GEOMETRIC_REPRESENTATION_CONTEXT(3)
GLOBAL_UNCERTAINTY_ASSIGNED_CONTEXT((#7782))
GLOBAL_UNIT_ASSIGNED_CONTEXT((#7807,#7809,#7810))
REPRESENTATION_CONTEXT('','3D')
);
#7807=(
LENGTH_UNIT()
NAMED_UNIT(*)
SI_UNIT(.CENTI.,.METRE.)
);
#7809=(
NAMED_UNIT(*)
PLANE_ANGLE_UNIT()
SI_UNIT($,.RADIAN.)
);
#7810=(
NAMED_UNIT(*)
SI_UNIT($,.STERADIAN.)
SOLID_ANGLE_UNIT()
);
#7813=SHAPE_DEFINITION_REPRESENTATION(#7836,#7912);
#7836=PRODUCT_DEFINITION_SHAPE('',$,#7936);
#7912=SHAPE_REPRESENTATION('',(#4428),#7785);
#7933=PRODUCT_DEFINITION_CONTEXT('part definition',#8004,'design');
#7936=PRODUCT_DEFINITION('Slotted Extrusion - 20 x 20 x 300 mm',
'Slotted Extrusion - 20 x 20 x 300 mm',#7959,#7933);
#7959=PRODUCT_DEFINITION_FORMATION('',$,#8008);
#8004=APPLICATION_CONTEXT(
'Core Data for Automotive Mechanical Design Process');
#8005=PRODUCT_CONTEXT('part definition',#8004,'mechanical');
#8008=PRODUCT('Slotted Extrusion - 20 x 20 x 300 mm',
'Slotted Extrusion - 20 x 20 x 300 mm',
'Slotted Extrusion - 20 x 20 x 300 mm',(#8005));
#8099=COLOUR_RGB('Off White',0.89,0.88,0.83);
#8100=FILL_AREA_STYLE_COLOUR('',#8099);
#8101=FILL_AREA_STYLE('',(#8100));
#8102=SURFACE_STYLE_FILL_AREA(#8101);
#8103=SURFACE_SIDE_STYLE('',(#8102));
#8104=SURFACE_STYLE_USAGE(.BOTH.,#8103);
#8105=PRESENTATION_STYLE_ASSIGNMENT((#8104));
ENDSEC;
END-ISO-10303-21;
